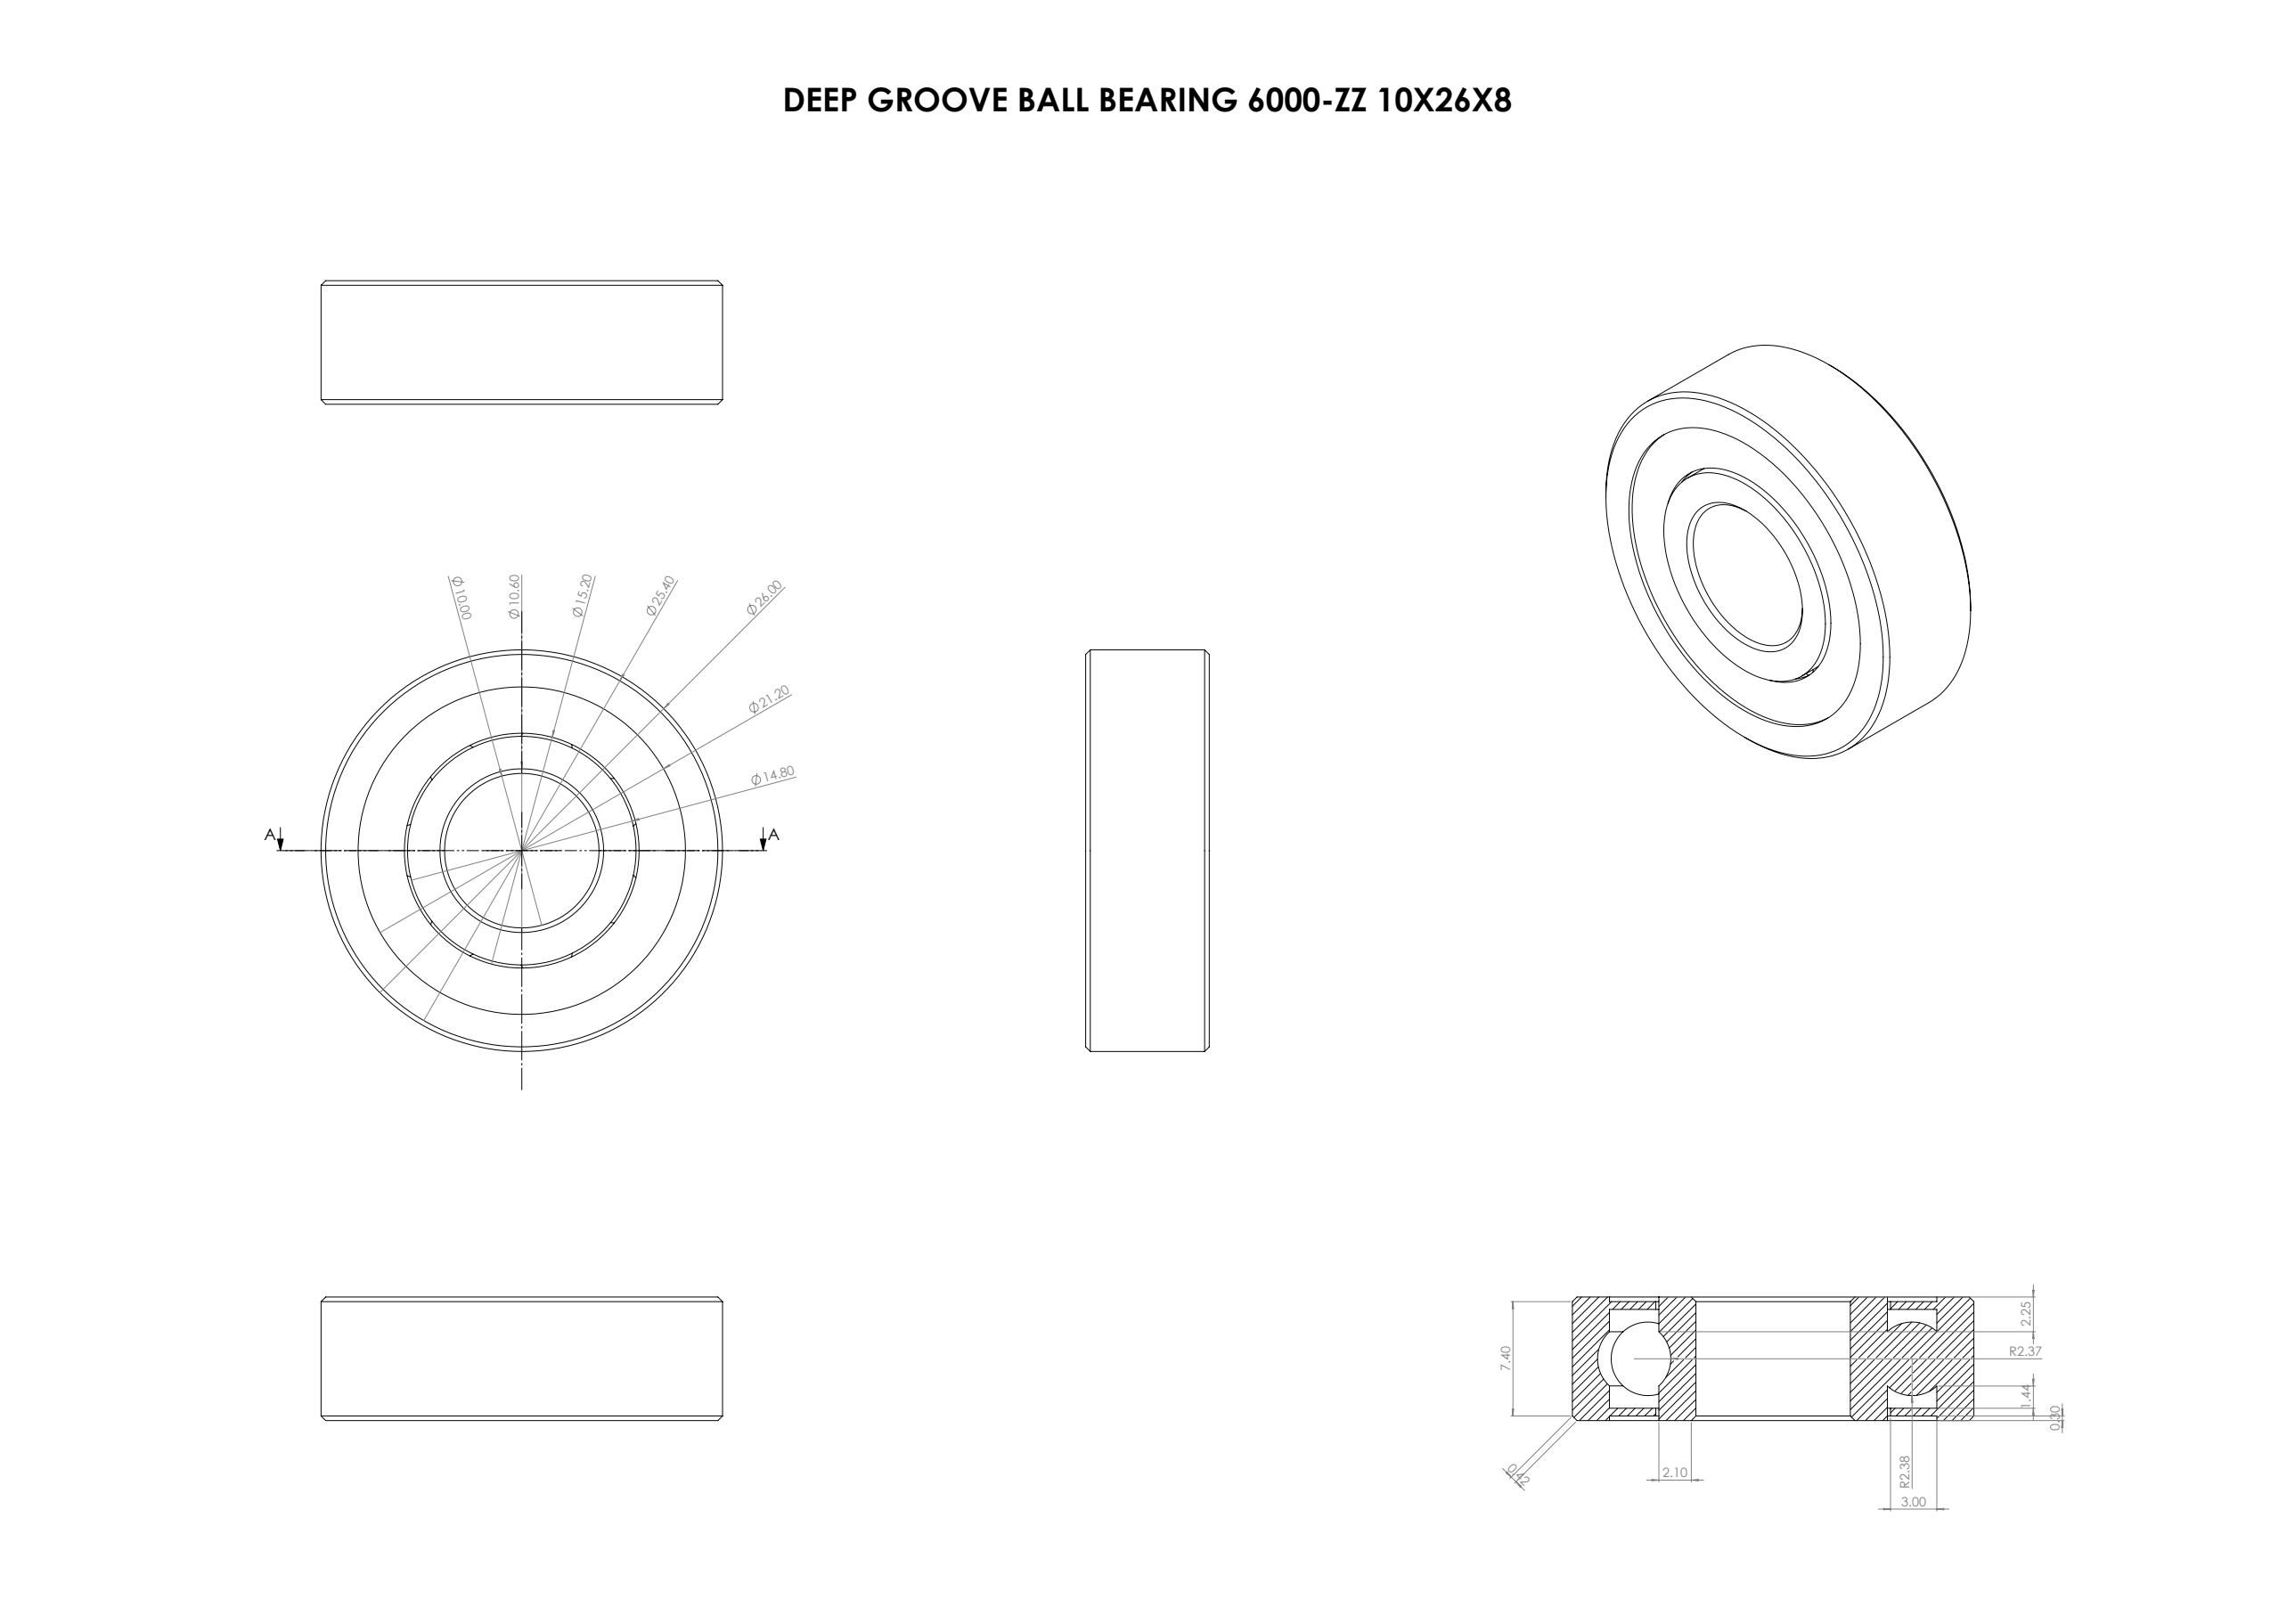
ISO-10303-21;
HEADER;
/* Generated by software containing ST-Developer
 * from STEP Tools, Inc. (www.steptools.com) 
 */

FILE_DESCRIPTION(
/* description */ (''),
/* implementation_level */ '2;1');

FILE_NAME(
/* name */ 
'05_Deep_Groove_Ball_Bearing_6000-ZZ_10x26x8.step',
/* time_stamp */ '2026-10-22T00:21:42-07:00',
/* author */ (''),
/* organization */ (''),
/* preprocessor_version */ 'ST-DEVELOPER v20.2',
/* originating_system */ 'Autodesk Translation Framework v15.15.0.0',
/* authorisation */ '');

FILE_SCHEMA (('AUTOMOTIVE_DESIGN { 1 0 10303 214 3 1 1 }'));
ENDSEC;

DATA;
#10=MECHANICAL_DESIGN_GEOMETRIC_PRESENTATION_REPRESENTATION('',(#209),#31638);
#176=SPHERICAL_SURFACE('',#13012,0.23815);
#177=SPHERICAL_SURFACE('',#13037,0.23815);
#178=SPHERICAL_SURFACE('',#13043,0.23815);
#179=SPHERICAL_SURFACE('',#13050,0.23815);
#180=SPHERICAL_SURFACE('',#13056,0.23815);
#181=SPHERICAL_SURFACE('',#13062,0.23815);
#182=SPHERICAL_SURFACE('',#13073,0.23815);
#187=SHAPE_REPRESENTATION_RELATIONSHIP('SRR','None',#31709,#198);
#198=ADVANCED_BREP_SHAPE_REPRESENTATION('',(#220),#31631);
#209=STYLED_ITEM('',(#31830),#220);
#220=MANIFOLD_SOLID_BREP('6000-ZZ rings + balls + shields',#12484);
#231=TOROIDAL_SURFACE('',#13024,0.9,0.2374);
#232=TOROIDAL_SURFACE('',#13035,0.9,0.2374);
#233=TOROIDAL_SURFACE('',#13040,0.9,0.2374);
#234=TOROIDAL_SURFACE('',#13041,0.9,0.2374);
#235=TOROIDAL_SURFACE('',#13046,0.9,0.2374);
#236=TOROIDAL_SURFACE('',#13047,0.9,0.2374);
#237=TOROIDAL_SURFACE('',#13053,0.9,0.2374);
#238=TOROIDAL_SURFACE('',#13054,0.9,0.2374);
#239=TOROIDAL_SURFACE('',#13059,0.9,0.2374);
#240=TOROIDAL_SURFACE('',#13060,0.9,0.2374);
#241=TOROIDAL_SURFACE('',#13067,0.9,0.2374);
#242=TOROIDAL_SURFACE('',#13072,0.9,0.2374);
#243=TOROIDAL_SURFACE('',#13076,0.9,0.2374);
#244=TOROIDAL_SURFACE('',#13086,0.9,0.2374);
#277=CYLINDRICAL_SURFACE('',#12993,0.76);
#278=CYLINDRICAL_SURFACE('',#12994,1.06);
#279=CYLINDRICAL_SURFACE('',#13002,0.76);
#280=CYLINDRICAL_SURFACE('',#13003,1.06);
#281=CYLINDRICAL_SURFACE('',#13015,1.06);
#282=CYLINDRICAL_SURFACE('',#13025,0.74);
#283=CYLINDRICAL_SURFACE('',#13065,1.06);
#284=CYLINDRICAL_SURFACE('',#13068,0.74);
#285=CYLINDRICAL_SURFACE('',#13081,1.3);
#286=CYLINDRICAL_SURFACE('',#13087,0.5);
#431=CONICAL_SURFACE('',#13079,1.285,0.785398163397452);
#432=CONICAL_SURFACE('',#13083,1.285,0.785398163397452);
#433=CONICAL_SURFACE('',#13090,0.515,0.785398163397452);
#434=CONICAL_SURFACE('',#13095,0.515,0.785398163397452);
#945=B_SPLINE_CURVE_WITH_KNOTS('',3,(#24703,#24704,#24705,#24706,#24707,
#24708),.UNSPECIFIED.,.F.,.F.,(4,2,4),(0.254797907722713,0.274731256245471,
0.294664604768228),.UNSPECIFIED.);
#946=B_SPLINE_CURVE_WITH_KNOTS('',3,(#24712,#24713,#24714,#24715,#24716,
#24717),.UNSPECIFIED.,.F.,.F.,(4,2,4),(0.254797907722713,0.274731256245471,
0.294664604768229),.UNSPECIFIED.);
#947=B_SPLINE_CURVE_WITH_KNOTS('',3,(#24721,#24722,#24723,#24724,#24725,
#24726),.UNSPECIFIED.,.F.,.F.,(4,2,4),(0.254797907722713,0.274731256245471,
0.294664604768229),.UNSPECIFIED.);
#948=B_SPLINE_CURVE_WITH_KNOTS('',3,(#24730,#24731,#24732,#24733,#24734,
#24735),.UNSPECIFIED.,.F.,.F.,(4,2,4),(0.254797907722713,0.274731256245471,
0.294664604768228),.UNSPECIFIED.);
#949=B_SPLINE_CURVE_WITH_KNOTS('',3,(#24739,#24740,#24741,#24742,#24743,
#24744),.UNSPECIFIED.,.F.,.F.,(4,2,4),(0.254797907722728,0.274731256245471,
0.294664604768213),.UNSPECIFIED.);
#950=B_SPLINE_CURVE_WITH_KNOTS('',3,(#24751,#24752,#24753,#24754,#24755,
#24756),.UNSPECIFIED.,.F.,.F.,(4,2,4),(0.254797907722713,0.274731256245471,
0.294664604768229),.UNSPECIFIED.);
#951=B_SPLINE_CURVE_WITH_KNOTS('',3,(#24760,#24761,#24762,#24763,#24764,
#24765),.UNSPECIFIED.,.F.,.F.,(4,2,4),(0.254797907722728,0.274731256245471,
0.294664604768213),.UNSPECIFIED.);
#952=B_SPLINE_CURVE_WITH_KNOTS('',3,(#24770,#24771,#24772,#24773),
 .UNSPECIFIED.,.F.,.F.,(4,4),(0.750997797800867,0.767662411819255),
 .UNSPECIFIED.);
#953=B_SPLINE_CURVE_WITH_KNOTS('',3,(#24775,#24776,#24777,#24778,#24779,
#24780,#24781,#24782,#24783,#24784,#24785,#24786,#24787,#24788,#24789,#24790,
#24791,#24792,#24793,#24794,#24795,#24796),.UNSPECIFIED.,.F.,.F.,(4,2,2,
2,2,2,2,2,2,2,4),(0.516725915130786,0.527390969880923,0.571339243451659,
0.615287517022395,0.659234130021226,0.703180743020057,0.747127356018888,
0.791073969017719,0.835022242588455,0.878970516159191,0.889635570909327),
 .UNSPECIFIED.);
#954=B_SPLINE_CURVE_WITH_KNOTS('',3,(#24798,#24799,#24800,#24801),
 .UNSPECIFIED.,.F.,.F.,(4,4),(0.255887470606418,0.272552084624806),
 .UNSPECIFIED.);
#955=B_SPLINE_CURVE_WITH_KNOTS('',3,(#24805,#24806,#24807,#24808),
 .UNSPECIFIED.,.F.,.F.,(4,4),(0.239222856588031,0.255887470606418),
 .UNSPECIFIED.);
#956=B_SPLINE_CURVE_WITH_KNOTS('',3,(#24810,#24811,#24812,#24813,#24814,
#24815,#24816,#24817,#24818,#24819,#24820,#24821,#24822,#24823,#24824,#24825,
#24826,#24827,#24828,#24829,#24830,#24831),.UNSPECIFIED.,.F.,.F.,(4,2,2,
2,2,2,2,2,2,2,4),(0.516725915130786,0.527390969880923,0.571339243451659,
0.615287517022395,0.659234130021226,0.703180743020057,0.747127356018888,
0.791073969017718,0.835022242588455,0.878970516159191,0.889635570909327),
 .UNSPECIFIED.);
#957=B_SPLINE_CURVE_WITH_KNOTS('',3,(#24832,#24833,#24834,#24835),
 .UNSPECIFIED.,.F.,.F.,(4,4),(0.767662411819255,0.784327025837643),
 .UNSPECIFIED.);
#958=B_SPLINE_CURVE_WITH_KNOTS('',3,(#24839,#24840,#24841,#24842,#24843,
#24844,#24845,#24846,#24847,#24848,#24849,#24850,#24851,#24852,#24853,#24854,
#24855,#24856,#24857,#24858,#24859,#24860,#24861),.UNSPECIFIED.,.F.,.F.,
(4,2,2,2,2,3,2,2,2,2,4),(-0.186453873187253,-0.17578960100413,-0.131841711164795,
-0.087893821325461,-0.0439469106627304,0.,0.0439469106627304,0.0878938213254609,
0.131841711164795,0.17578960100413,0.186453873187381),.UNSPECIFIED.);
#959=B_SPLINE_CURVE_WITH_KNOTS('',3,(#24863,#24864,#24865,#24866,#24867,
#24868),.UNSPECIFIED.,.F.,.F.,(4,2,4),(0.804260420213654,0.824193768736411,
0.844127117259169),.UNSPECIFIED.);
#960=B_SPLINE_CURVE_WITH_KNOTS('',3,(#24869,#24870,#24871,#24872,#24873,
#24874,#24875,#24876,#24877,#24878,#24879,#24880,#24881,#24882,#24883,#24884,
#24885,#24886,#24887,#24888,#24889,#24890,#24891),.UNSPECIFIED.,.F.,.F.,
(4,2,2,2,2,3,2,2,2,2,4),(-0.186453873187253,-0.17578960100413,-0.131841711164795,
-0.087893821325461,-0.0439469106627306,0.,0.0439469106627304,0.0878938213254609,
0.131841711164795,0.17578960100413,0.186453873187381),.UNSPECIFIED.);
#961=B_SPLINE_CURVE_WITH_KNOTS('',3,(#24898,#24899,#24900,#24901,#24902,
#24903),.UNSPECIFIED.,.F.,.F.,(4,2,4),(0.804260420213644,0.824193768736412,
0.84412711725918),.UNSPECIFIED.);
#962=B_SPLINE_CURVE_WITH_KNOTS('',3,(#24907,#24908,#24909,#24910,#24911,
#24912),.UNSPECIFIED.,.F.,.F.,(4,2,4),(0.804260420213654,0.824193768736412,
0.84412711725917),.UNSPECIFIED.);
#963=B_SPLINE_CURVE_WITH_KNOTS('',3,(#24916,#24917,#24918,#24919,#24920,
#24921),.UNSPECIFIED.,.F.,.F.,(4,2,4),(0.804260420213654,0.824193768736411,
0.844127117259169),.UNSPECIFIED.);
#964=B_SPLINE_CURVE_WITH_KNOTS('',3,(#24925,#24926,#24927,#24928,#24929,
#24930),.UNSPECIFIED.,.F.,.F.,(4,2,4),(0.804260420213654,0.824193768736411,
0.844127117259169),.UNSPECIFIED.);
#965=B_SPLINE_CURVE_WITH_KNOTS('',3,(#24935,#24936,#24937,#24938,#24939,
#24940),.UNSPECIFIED.,.F.,.F.,(4,2,4),(0.804260420213643,0.824193768736411,
0.844127117259179),.UNSPECIFIED.);
#966=B_SPLINE_CURVE_WITH_KNOTS('',3,(#24944,#24945,#24946,#24947,#24948,
#24949),.UNSPECIFIED.,.F.,.F.,(4,2,4),(0.804260420213654,0.824193768736412,
0.844127117259169),.UNSPECIFIED.);
#967=B_SPLINE_CURVE_WITH_KNOTS('',3,(#24952,#24953,#24954,#24955,#24956,
#24957,#24958,#24959,#24960,#24961,#24962,#24963,#24964,#24965,#24966,#24967,
#24968,#24969,#24970,#24971,#24972,#24973,#24974),.UNSPECIFIED.,.F.,.F.,
(4,2,2,2,2,3,2,2,2,2,4),(-0.186453873187254,-0.17578960100413,-0.131841711164795,
-0.087893821325461,-0.0439469106627304,0.,0.0439469106627307,0.0878938213254614,
0.131841711164796,0.17578960100413,0.186453873187382),.UNSPECIFIED.);
#968=B_SPLINE_CURVE_WITH_KNOTS('',3,(#24979,#24980,#24981,#24982),
 .UNSPECIFIED.,.F.,.F.,(4,4),(0.23922285658804,0.255887470606418),
 .UNSPECIFIED.);
#969=B_SPLINE_CURVE_WITH_KNOTS('',3,(#24984,#24985,#24986,#24987),
 .UNSPECIFIED.,.F.,.F.,(4,4),(0.255887470606418,0.272552084624797),
 .UNSPECIFIED.);
#970=B_SPLINE_CURVE_WITH_KNOTS('',3,(#24991,#24992,#24993,#24994),
 .UNSPECIFIED.,.F.,.F.,(4,4),(0.239222856588031,0.255887470606418),
 .UNSPECIFIED.);
#971=B_SPLINE_CURVE_WITH_KNOTS('',3,(#24996,#24997,#24998,#24999),
 .UNSPECIFIED.,.F.,.F.,(4,4),(0.255887470606418,0.272552084624806),
 .UNSPECIFIED.);
#972=B_SPLINE_CURVE_WITH_KNOTS('',3,(#25008,#25009,#25010,#25011),
 .UNSPECIFIED.,.F.,.F.,(4,4),(0.239222856588039,0.255887470606418),
 .UNSPECIFIED.);
#973=B_SPLINE_CURVE_WITH_KNOTS('',3,(#25013,#25014,#25015,#25016),
 .UNSPECIFIED.,.F.,.F.,(4,4),(0.255887470606418,0.272552084624797),
 .UNSPECIFIED.);
#974=B_SPLINE_CURVE_WITH_KNOTS('',3,(#25020,#25021,#25022,#25023),
 .UNSPECIFIED.,.F.,.F.,(4,4),(0.239222856588031,0.255887470606418),
 .UNSPECIFIED.);
#975=B_SPLINE_CURVE_WITH_KNOTS('',3,(#25025,#25026,#25027,#25028),
 .UNSPECIFIED.,.F.,.F.,(4,4),(0.255887470606418,0.272552084624806),
 .UNSPECIFIED.);
#976=B_SPLINE_CURVE_WITH_KNOTS('',3,(#25032,#25033,#25034,#25035),
 .UNSPECIFIED.,.F.,.F.,(4,4),(0.239222856588031,0.255887470606418),
 .UNSPECIFIED.);
#977=B_SPLINE_CURVE_WITH_KNOTS('',3,(#25037,#25038,#25039,#25040),
 .UNSPECIFIED.,.F.,.F.,(4,4),(0.255887470606418,0.272552084624806),
 .UNSPECIFIED.);
#978=B_SPLINE_CURVE_WITH_KNOTS('',3,(#25044,#25045,#25046,#25047),
 .UNSPECIFIED.,.F.,.F.,(4,4),(0.239222856588031,0.255887470606418),
 .UNSPECIFIED.);
#979=B_SPLINE_CURVE_WITH_KNOTS('',3,(#25049,#25050,#25051,#25052),
 .UNSPECIFIED.,.F.,.F.,(4,4),(0.255887470606418,0.272552084624806),
 .UNSPECIFIED.);
#980=B_SPLINE_CURVE_WITH_KNOTS('',3,(#25057,#25058,#25059,#25060,#25061,
#25062,#25063,#25064,#25065,#25066,#25067,#25068,#25069,#25070,#25071,#25072,
#25073,#25074,#25075,#25076,#25077,#25078),.UNSPECIFIED.,.F.,.F.,(4,2,2,
2,2,2,2,2,2,2,4),(0.516725915130786,0.527390969880923,0.571339243451659,
0.615287517022395,0.659234130021226,0.703180743020057,0.747127356018888,
0.791073969017719,0.835022242588455,0.878970516159191,0.889635570909327),
 .UNSPECIFIED.);
#981=B_SPLINE_CURVE_WITH_KNOTS('',3,(#25082,#25083,#25084,#25085),
 .UNSPECIFIED.,.F.,.F.,(4,4),(0.750997797800864,0.767662411819255),
 .UNSPECIFIED.);
#982=B_SPLINE_CURVE_WITH_KNOTS('',3,(#25086,#25087,#25088,#25089,#25090,
#25091,#25092,#25093,#25094,#25095,#25096,#25097,#25098,#25099,#25100,#25101,
#25102,#25103,#25104,#25105,#25106,#25107),.UNSPECIFIED.,.F.,.F.,(4,2,2,
2,2,2,2,2,2,2,4),(0.516725915130786,0.527390969880923,0.571339243451659,
0.615287517022395,0.659234130021226,0.703180743020056,0.747127356018887,
0.791073969017719,0.835022242588454,0.87897051615919,0.889635570909327),
 .UNSPECIFIED.);
#983=B_SPLINE_CURVE_WITH_KNOTS('',3,(#25110,#25111,#25112,#25113),
 .UNSPECIFIED.,.F.,.F.,(4,4),(0.767662411819255,0.784327025837645),
 .UNSPECIFIED.);
#984=B_SPLINE_CURVE_WITH_KNOTS('',3,(#25116,#25117,#25118,#25119,#25120,
#25121,#25122,#25123,#25124,#25125,#25126,#25127,#25128,#25129,#25130,#25131,
#25132,#25133,#25134,#25135,#25136,#25137,#25138),.UNSPECIFIED.,.F.,.F.,
(4,2,2,2,2,3,2,2,2,2,4),(-0.186453873187254,-0.17578960100413,-0.131841711164796,
-0.0878938213254614,-0.0439469106627306,0.,0.0439469106627305,0.0878938213254609,
0.131841711164795,0.175789601004129,0.186453873187382),.UNSPECIFIED.);
#985=B_SPLINE_CURVE_WITH_KNOTS('',3,(#25140,#25141,#25142,#25143,#25144,
#25145,#25146,#25147,#25148,#25149,#25150,#25151,#25152,#25153,#25154,#25155,
#25156,#25157,#25158,#25159,#25160,#25161,#25162),.UNSPECIFIED.,.F.,.F.,
(4,2,2,2,2,3,2,2,2,2,4),(-0.186453873187253,-0.17578960100413,-0.131841711164795,
-0.087893821325461,-0.0439469106627306,0.,0.0439469106627305,0.0878938213254609,
0.131841711164795,0.17578960100413,0.186453873187381),.UNSPECIFIED.);
#986=B_SPLINE_CURVE_WITH_KNOTS('',3,(#25166,#25167,#25168,#25169,#25170,
#25171,#25172,#25173,#25174,#25175,#25176,#25177,#25178,#25179,#25180,#25181,
#25182,#25183,#25184,#25185,#25186,#25187),.UNSPECIFIED.,.F.,.F.,(4,2,2,
2,2,2,2,2,2,2,4),(0.516725915130786,0.527390969880923,0.571339243451659,
0.615287517022395,0.659234130021226,0.703180743020057,0.747127356018888,
0.791073969017718,0.835022242588455,0.878970516159191,0.889635570909327),
 .UNSPECIFIED.);
#987=B_SPLINE_CURVE_WITH_KNOTS('',3,(#25191,#25192,#25193,#25194),
 .UNSPECIFIED.,.F.,.F.,(4,4),(0.750997797800867,0.767662411819255),
 .UNSPECIFIED.);
#988=B_SPLINE_CURVE_WITH_KNOTS('',3,(#25195,#25196,#25197,#25198,#25199,
#25200,#25201,#25202,#25203,#25204,#25205,#25206,#25207,#25208,#25209,#25210,
#25211,#25212,#25213,#25214,#25215,#25216),.UNSPECIFIED.,.F.,.F.,(4,2,2,
2,2,2,2,2,2,2,4),(0.516725915130786,0.527390969880923,0.571339243451659,
0.615287517022395,0.659234130021226,0.703180743020057,0.747127356018888,
0.791073969017718,0.835022242588454,0.87897051615919,0.889635570909327),
 .UNSPECIFIED.);
#989=B_SPLINE_CURVE_WITH_KNOTS('',3,(#25219,#25220,#25221,#25222),
 .UNSPECIFIED.,.F.,.F.,(4,4),(0.767662411819255,0.784327025837642),
 .UNSPECIFIED.);
#990=B_SPLINE_CURVE_WITH_KNOTS('',3,(#25225,#25226,#25227,#25228,#25229,
#25230,#25231,#25232,#25233,#25234,#25235,#25236,#25237,#25238,#25239,#25240,
#25241,#25242,#25243,#25244,#25245,#25246,#25247),.UNSPECIFIED.,.F.,.F.,
(4,2,2,2,2,3,2,2,2,2,4),(-0.186453873187253,-0.17578960100413,-0.131841711164795,
-0.0878938213254608,-0.0439469106627304,0.,0.0439469106627304,0.0878938213254609,
0.131841711164795,0.17578960100413,0.186453873187381),.UNSPECIFIED.);
#991=B_SPLINE_CURVE_WITH_KNOTS('',3,(#25249,#25250,#25251,#25252,#25253,
#25254,#25255,#25256,#25257,#25258,#25259,#25260,#25261,#25262,#25263,#25264,
#25265,#25266,#25267,#25268,#25269,#25270,#25271),.UNSPECIFIED.,.F.,.F.,
(4,2,2,2,2,3,2,2,2,2,4),(-0.186453873187254,-0.17578960100413,-0.131841711164796,
-0.0878938213254614,-0.0439469106627308,0.,0.0439469106627309,0.0878938213254618,
0.131841711164796,0.17578960100413,0.186453873187382),.UNSPECIFIED.);
#992=B_SPLINE_CURVE_WITH_KNOTS('',3,(#25277,#25278,#25279,#25280,#25281,
#25282,#25283,#25284,#25285,#25286,#25287,#25288,#25289,#25290,#25291,#25292,
#25293,#25294,#25295,#25296,#25297,#25298),.UNSPECIFIED.,.F.,.F.,(4,2,2,
2,2,2,2,2,2,2,4),(0.516725915130787,0.527390969880924,0.571339243451659,
0.615287517022395,0.659234130021226,0.703180743020058,0.747127356018888,
0.791073969017719,0.835022242588455,0.878970516159191,0.889635570909328),
 .UNSPECIFIED.);
#993=B_SPLINE_CURVE_WITH_KNOTS('',3,(#25302,#25303,#25304,#25305),
 .UNSPECIFIED.,.F.,.F.,(4,4),(0.750997797800863,0.767662411819254),
 .UNSPECIFIED.);
#994=B_SPLINE_CURVE_WITH_KNOTS('',3,(#25306,#25307,#25308,#25309,#25310,
#25311,#25312,#25313,#25314,#25315,#25316,#25317,#25318,#25319,#25320,#25321,
#25322,#25323,#25324,#25325,#25326,#25327),.UNSPECIFIED.,.F.,.F.,(4,2,2,
2,2,2,2,2,2,2,4),(0.516725915130786,0.527390969880923,0.571339243451659,
0.615287517022395,0.659234130021226,0.703180743020056,0.747127356018888,
0.791073969017719,0.835022242588455,0.87897051615919,0.889635570909327),
 .UNSPECIFIED.);
#995=B_SPLINE_CURVE_WITH_KNOTS('',3,(#25330,#25331,#25332,#25333),
 .UNSPECIFIED.,.F.,.F.,(4,4),(0.767662411819254,0.784327025837645),
 .UNSPECIFIED.);
#996=B_SPLINE_CURVE_WITH_KNOTS('',3,(#25336,#25337,#25338,#25339,#25340,
#25341,#25342,#25343,#25344,#25345,#25346,#25347,#25348,#25349,#25350,#25351,
#25352,#25353,#25354,#25355,#25356,#25357,#25358),.UNSPECIFIED.,.F.,.F.,
(4,2,2,2,2,3,2,2,2,2,4),(-0.186453873187254,-0.17578960100413,-0.131841711164796,
-0.0878938213254616,-0.0439469106627308,0.,0.0439469106627307,0.0878938213254613,
0.131841711164795,0.17578960100413,0.186453873187382),.UNSPECIFIED.);
#997=B_SPLINE_CURVE_WITH_KNOTS('',3,(#25360,#25361,#25362,#25363,#25364,
#25365,#25366,#25367,#25368,#25369,#25370,#25371,#25372,#25373,#25374,#25375,
#25376,#25377,#25378,#25379,#25380,#25381,#25382),.UNSPECIFIED.,.F.,.F.,
(4,2,2,2,2,3,2,2,2,2,4),(-0.186453873187253,-0.17578960100413,-0.131841711164795,
-0.0878938213254608,-0.0439469106627304,0.,0.0439469106627304,0.0878938213254609,
0.131841711164795,0.17578960100413,0.186453873187382),.UNSPECIFIED.);
#998=B_SPLINE_CURVE_WITH_KNOTS('',3,(#25386,#25387,#25388,#25389,#25390,
#25391,#25392,#25393,#25394,#25395,#25396,#25397,#25398,#25399,#25400,#25401,
#25402,#25403,#25404,#25405,#25406,#25407),.UNSPECIFIED.,.F.,.F.,(4,2,2,
2,2,2,2,2,2,2,4),(0.516725915130786,0.527390969880923,0.571339243451659,
0.615287517022395,0.659234130021226,0.703180743020057,0.747127356018888,
0.791073969017719,0.835022242588455,0.878970516159191,0.889635570909327),
 .UNSPECIFIED.);
#999=B_SPLINE_CURVE_WITH_KNOTS('',3,(#25411,#25412,#25413,#25414),
 .UNSPECIFIED.,.F.,.F.,(4,4),(0.750997797800867,0.767662411819255),
 .UNSPECIFIED.);
#1000=B_SPLINE_CURVE_WITH_KNOTS('',3,(#25415,#25416,#25417,#25418,#25419,
#25420,#25421,#25422,#25423,#25424,#25425,#25426,#25427,#25428,#25429,#25430,
#25431,#25432,#25433,#25434,#25435,#25436),.UNSPECIFIED.,.F.,.F.,(4,2,2,
2,2,2,2,2,2,2,4),(0.516725915130786,0.527390969880923,0.571339243451659,
0.615287517022395,0.659234130021226,0.703180743020057,0.747127356018888,
0.791073969017718,0.835022242588454,0.87897051615919,0.889635570909327),
 .UNSPECIFIED.);
#1001=B_SPLINE_CURVE_WITH_KNOTS('',3,(#25439,#25440,#25441,#25442),
 .UNSPECIFIED.,.F.,.F.,(4,4),(0.767662411819255,0.784327025837643),
 .UNSPECIFIED.);
#1002=B_SPLINE_CURVE_WITH_KNOTS('',3,(#25445,#25446,#25447,#25448,#25449,
#25450,#25451,#25452,#25453,#25454,#25455,#25456,#25457,#25458,#25459,#25460,
#25461,#25462,#25463,#25464,#25465,#25466,#25467),.UNSPECIFIED.,.F.,.F.,
(4,2,2,2,2,3,2,2,2,2,4),(-0.186453873187253,-0.17578960100413,-0.131841711164795,
-0.0878938213254608,-0.0439469106627304,0.,0.0439469106627304,0.0878938213254608,
0.131841711164795,0.17578960100413,0.186453873187381),.UNSPECIFIED.);
#1003=B_SPLINE_CURVE_WITH_KNOTS('',3,(#25469,#25470,#25471,#25472,#25473,
#25474,#25475,#25476,#25477,#25478,#25479,#25480,#25481,#25482,#25483,#25484,
#25485,#25486,#25487,#25488,#25489,#25490,#25491),.UNSPECIFIED.,.F.,.F.,
(4,2,2,2,2,3,2,2,2,2,4),(-0.186453873187253,-0.17578960100413,-0.131841711164796,
-0.0878938213254616,-0.0439469106627308,0.,0.0439469106627304,0.0878938213254609,
0.131841711164795,0.17578960100413,0.186453873187382),.UNSPECIFIED.);
#1004=B_SPLINE_CURVE_WITH_KNOTS('',3,(#25495,#25496,#25497,#25498,#25499,
#25500,#25501,#25502,#25503,#25504,#25505,#25506,#25507,#25508,#25509,#25510,
#25511,#25512,#25513,#25514,#25515,#25516),.UNSPECIFIED.,.F.,.F.,(4,2,2,
2,2,2,2,2,2,2,4),(0.516725915130786,0.527390969880923,0.571339243451659,
0.615287517022395,0.659234130021226,0.703180743020057,0.747127356018888,
0.791073969017719,0.835022242588455,0.878970516159191,0.889635570909328),
 .UNSPECIFIED.);
#1005=B_SPLINE_CURVE_WITH_KNOTS('',3,(#25519,#25520,#25521,#25522),
 .UNSPECIFIED.,.F.,.F.,(4,4),(0.767662411819255,0.784327025837642),
 .UNSPECIFIED.);
#1006=B_SPLINE_CURVE_WITH_KNOTS('',3,(#25526,#25527,#25528,#25529),
 .UNSPECIFIED.,.F.,.F.,(4,4),(0.750997797800867,0.767662411819255),
 .UNSPECIFIED.);
#1007=B_SPLINE_CURVE_WITH_KNOTS('',3,(#25530,#25531,#25532,#25533,#25534,
#25535,#25536,#25537,#25538,#25539,#25540,#25541,#25542,#25543,#25544,#25545,
#25546,#25547,#25548,#25549,#25550,#25551),.UNSPECIFIED.,.F.,.F.,(4,2,2,
2,2,2,2,2,2,2,4),(0.516725915130786,0.527390969880923,0.571339243451659,
0.615287517022395,0.659234130021226,0.703180743020057,0.747127356018888,
0.791073969017719,0.835022242588455,0.878970516159191,0.889635570909327),
 .UNSPECIFIED.);
#1008=B_SPLINE_CURVE_WITH_KNOTS('',3,(#25554,#25555,#25556,#25557,#25558,
#25559,#25560,#25561,#25562,#25563,#25564,#25565,#25566,#25567,#25568,#25569,
#25570,#25571,#25572,#25573,#25574,#25575,#25576),.UNSPECIFIED.,.F.,.F.,
(4,2,2,2,2,3,2,2,2,2,4),(-0.186453873187254,-0.17578960100413,-0.131841711164795,
-0.087893821325461,-0.0439469106627304,0.,0.0439469106627308,0.0878938213254617,
0.131841711164796,0.17578960100413,0.186453873187381),.UNSPECIFIED.);
#1009=B_SPLINE_CURVE_WITH_KNOTS('',3,(#25582,#25583,#25584,#25585,#25586,
#25587,#25588,#25589,#25590,#25591,#25592,#25593,#25594,#25595,#25596,#25597,
#25598,#25599,#25600,#25601,#25602,#25603,#25604),.UNSPECIFIED.,.F.,.F.,
(4,2,2,2,2,3,2,2,2,2,4),(-0.186453873187253,-0.17578960100413,-0.131841711164795,
-0.0878938213254608,-0.0439469106627304,0.,0.0439469106627304,0.0878938213254609,
0.131841711164795,0.17578960100413,0.186453873187381),.UNSPECIFIED.);
#1010=B_SPLINE_CURVE_WITH_KNOTS('',3,(#25612,#25613,#25614,#25615),
 .UNSPECIFIED.,.F.,.F.,(4,4),(0.750997797800867,0.767662411819255),
 .UNSPECIFIED.);
#1011=B_SPLINE_CURVE_WITH_KNOTS('',3,(#25617,#25618,#25619,#25620),
 .UNSPECIFIED.,.F.,.F.,(4,4),(0.767662411819255,0.784327025837643),
 .UNSPECIFIED.);
#1012=B_SPLINE_CURVE_WITH_KNOTS('',3,(#25623,#25624,#25625,#25626,#25627,
#25628,#25629,#25630,#25631,#25632,#25633,#25634,#25635,#25636,#25637,#25638,
#25639,#25640,#25641,#25642,#25643,#25644),.UNSPECIFIED.,.F.,.F.,(4,2,2,
2,2,2,2,2,2,2,4),(0.516725915130786,0.527390969880923,0.571339243451659,
0.615287517022395,0.659234130021226,0.703180743020057,0.747127356018888,
0.791073969017719,0.835022242588455,0.878970516159191,0.889635570909328),
 .UNSPECIFIED.);
#1013=B_SPLINE_CURVE_WITH_KNOTS('',3,(#25648,#25649,#25650,#25651,#25652,
#25653,#25654,#25655,#25656,#25657,#25658,#25659,#25660,#25661,#25662,#25663,
#25664,#25665,#25666,#25667,#25668,#25669),.UNSPECIFIED.,.F.,.F.,(4,2,2,
2,2,2,2,2,2,2,4),(0.516725915130786,0.527390969880923,0.571339243451659,
0.615287517022395,0.659234130021226,0.703180743020057,0.747127356018888,
0.791073969017719,0.835022242588455,0.878970516159191,0.889635570909327),
 .UNSPECIFIED.);
#1014=B_SPLINE_CURVE_WITH_KNOTS('',3,(#25672,#25673,#25674,#25675,#25676,
#25677,#25678,#25679,#25680,#25681,#25682,#25683,#25684,#25685,#25686,#25687,
#25688,#25689,#25690,#25691,#25692,#25693,#25694),.UNSPECIFIED.,.F.,.F.,
(4,2,2,2,2,3,2,2,2,2,4),(-0.186453873187253,-0.17578960100413,-0.131841711164795,
-0.087893821325461,-0.0439469106627306,0.,0.0439469106627304,0.0878938213254609,
0.131841711164795,0.17578960100413,0.186453873187381),.UNSPECIFIED.);
#1375=FACE_BOUND('',#2887,.T.);
#1376=FACE_BOUND('',#2889,.T.);
#1377=FACE_BOUND('',#2893,.T.);
#1378=FACE_BOUND('',#2895,.T.);
#1379=FACE_BOUND('',#2899,.T.);
#1380=FACE_BOUND('',#2905,.T.);
#1381=FACE_BOUND('',#2909,.T.);
#1382=FACE_BOUND('',#2913,.T.);
#1383=FACE_BOUND('',#2917,.T.);
#1384=FACE_BOUND('',#2921,.T.);
#1385=FACE_BOUND('',#2927,.T.);
#1386=FACE_BOUND('',#2930,.T.);
#1387=FACE_BOUND('',#2935,.T.);
#1388=FACE_BOUND('',#2940,.T.);
#1389=FACE_BOUND('',#2942,.T.);
#1579=CIRCLE('',#12988,1.06);
#1580=CIRCLE('',#12989,0.76);
#1581=CIRCLE('',#12991,1.06);
#1582=CIRCLE('',#12992,0.76);
#1583=CIRCLE('',#12995,1.06);
#1584=CIRCLE('',#12997,1.06);
#1585=CIRCLE('',#12998,0.76);
#1586=CIRCLE('',#13000,1.06);
#1587=CIRCLE('',#13001,0.76);
#1588=CIRCLE('',#13004,1.06);
#1589=CIRCLE('',#13005,1.06);
#1590=CIRCLE('',#13006,1.06);
#1591=CIRCLE('',#13007,1.06);
#1592=CIRCLE('',#13008,1.06);
#1593=CIRCLE('',#13009,1.06);
#1594=CIRCLE('',#13010,1.06);
#1595=CIRCLE('',#13011,1.06);
#1596=CIRCLE('',#13013,0.23815);
#1597=CIRCLE('',#13014,0.23815);
#1598=CIRCLE('',#13016,1.06);
#1599=CIRCLE('',#13017,1.06);
#1600=CIRCLE('',#13018,1.06);
#1601=CIRCLE('',#13019,1.06);
#1602=CIRCLE('',#13020,1.06);
#1603=CIRCLE('',#13021,1.06);
#1604=CIRCLE('',#13022,1.06);
#1605=CIRCLE('',#13023,1.06);
#1606=CIRCLE('',#13026,0.74);
#1607=CIRCLE('',#13027,0.74);
#1608=CIRCLE('',#13028,0.74);
#1609=CIRCLE('',#13029,0.74);
#1610=CIRCLE('',#13030,0.74);
#1611=CIRCLE('',#13031,0.74);
#1612=CIRCLE('',#13032,0.74);
#1613=CIRCLE('',#13033,0.74);
#1614=CIRCLE('',#13034,0.74);
#1615=CIRCLE('',#13036,0.74);
#1616=CIRCLE('',#13038,0.23815);
#1617=CIRCLE('',#13039,0.23815);
#1618=CIRCLE('',#13042,0.74);
#1619=CIRCLE('',#13044,0.23815);
#1620=CIRCLE('',#13045,0.23815);
#1621=CIRCLE('',#13048,0.74);
#1622=CIRCLE('',#13049,0.74);
#1623=CIRCLE('',#13051,0.23815);
#1624=CIRCLE('',#13052,0.23815);
#1625=CIRCLE('',#13055,0.74);
#1626=CIRCLE('',#13057,0.23815);
#1627=CIRCLE('',#13058,0.23815);
#1628=CIRCLE('',#13061,0.74);
#1629=CIRCLE('',#13063,0.23815);
#1630=CIRCLE('',#13064,0.23815);
#1631=CIRCLE('',#13066,1.06);
#1632=CIRCLE('',#13069,0.74);
#1633=CIRCLE('',#13070,0.74);
#1634=CIRCLE('',#13071,0.74);
#1635=CIRCLE('',#13074,0.23815);
#1636=CIRCLE('',#13075,0.23815);
#1637=CIRCLE('',#13078,1.27);
#1638=CIRCLE('',#13080,1.3);
#1639=CIRCLE('',#13082,1.3);
#1640=CIRCLE('',#13084,1.27);
#1641=CIRCLE('',#13088,0.5);
#1642=CIRCLE('',#13089,0.5);
#1643=CIRCLE('',#13091,0.53);
#1644=CIRCLE('',#13094,0.53);
#2157=FACE_OUTER_BOUND('',#2886,.T.);
#2158=FACE_OUTER_BOUND('',#2888,.T.);
#2159=FACE_OUTER_BOUND('',#2890,.T.);
#2160=FACE_OUTER_BOUND('',#2891,.T.);
#2161=FACE_OUTER_BOUND('',#2892,.T.);
#2162=FACE_OUTER_BOUND('',#2894,.T.);
#2163=FACE_OUTER_BOUND('',#2896,.T.);
#2164=FACE_OUTER_BOUND('',#2897,.T.);
#2165=FACE_OUTER_BOUND('',#2898,.T.);
#2166=FACE_OUTER_BOUND('',#2900,.T.);
#2167=FACE_OUTER_BOUND('',#2901,.T.);
#2168=FACE_OUTER_BOUND('',#2902,.T.);
#2169=FACE_OUTER_BOUND('',#2903,.T.);
#2170=FACE_OUTER_BOUND('',#2904,.T.);
#2171=FACE_OUTER_BOUND('',#2906,.T.);
#2172=FACE_OUTER_BOUND('',#2907,.T.);
#2173=FACE_OUTER_BOUND('',#2908,.T.);
#2174=FACE_OUTER_BOUND('',#2910,.T.);
#2175=FACE_OUTER_BOUND('',#2911,.T.);
#2176=FACE_OUTER_BOUND('',#2912,.T.);
#2177=FACE_OUTER_BOUND('',#2914,.T.);
#2178=FACE_OUTER_BOUND('',#2915,.T.);
#2179=FACE_OUTER_BOUND('',#2916,.T.);
#2180=FACE_OUTER_BOUND('',#2918,.T.);
#2181=FACE_OUTER_BOUND('',#2919,.T.);
#2182=FACE_OUTER_BOUND('',#2920,.T.);
#2183=FACE_OUTER_BOUND('',#2922,.T.);
#2184=FACE_OUTER_BOUND('',#2923,.T.);
#2185=FACE_OUTER_BOUND('',#2924,.T.);
#2186=FACE_OUTER_BOUND('',#2925,.T.);
#2187=FACE_OUTER_BOUND('',#2926,.T.);
#2188=FACE_OUTER_BOUND('',#2928,.T.);
#2189=FACE_OUTER_BOUND('',#2929,.T.);
#2190=FACE_OUTER_BOUND('',#2931,.T.);
#2191=FACE_OUTER_BOUND('',#2932,.T.);
#2192=FACE_OUTER_BOUND('',#2933,.T.);
#2193=FACE_OUTER_BOUND('',#2934,.T.);
#2194=FACE_OUTER_BOUND('',#2936,.T.);
#2195=FACE_OUTER_BOUND('',#2937,.T.);
#2196=FACE_OUTER_BOUND('',#2938,.T.);
#2197=FACE_OUTER_BOUND('',#2939,.T.);
#2198=FACE_OUTER_BOUND('',#2941,.T.);
#2199=FACE_OUTER_BOUND('',#2943,.T.);
#2886=EDGE_LOOP('',(#9609));
#2887=EDGE_LOOP('',(#9610));
#2888=EDGE_LOOP('',(#9611));
#2889=EDGE_LOOP('',(#9612));
#2890=EDGE_LOOP('',(#9613,#9614,#9615,#9616));
#2891=EDGE_LOOP('',(#9617,#9618,#9619,#9620));
#2892=EDGE_LOOP('',(#9621));
#2893=EDGE_LOOP('',(#9622));
#2894=EDGE_LOOP('',(#9623));
#2895=EDGE_LOOP('',(#9624));
#2896=EDGE_LOOP('',(#9625,#9626,#9627,#9628));
#2897=EDGE_LOOP('',(#9629,#9630,#9631,#9632,#9633,#9634,#9635,#9636,#9637,
#9638,#9639,#9640,#9641,#9642,#9643,#9644,#9645,#9646));
#2898=EDGE_LOOP('',(#9647,#9648,#9649,#9650,#9651,#9652,#9653,#9654,#9655,
#9656));
#2899=EDGE_LOOP('',(#9657,#9658,#9659,#9660));
#2900=EDGE_LOOP('',(#9661,#9662,#9663,#9664,#9665,#9666,#9667,#9668,#9669,
#9670,#9671,#9672,#9673,#9674,#9675,#9676,#9677,#9678));
#2901=EDGE_LOOP('',(#9679,#9680,#9681,#9682));
#2902=EDGE_LOOP('',(#9683,#9684,#9685,#9686,#9687,#9688,#9689,#9690,#9691,
#9692,#9693,#9694,#9695,#9696,#9697,#9698,#9699,#9700,#9701,#9702,#9703,
#9704,#9705,#9706,#9707));
#2903=EDGE_LOOP('',(#9708,#9709,#9710,#9711));
#2904=EDGE_LOOP('',(#9712,#9713,#9714,#9715,#9716,#9717,#9718,#9719,#9720,
#9721));
#2905=EDGE_LOOP('',(#9722,#9723,#9724,#9725));
#2906=EDGE_LOOP('',(#9726,#9727,#9728,#9729));
#2907=EDGE_LOOP('',(#9730,#9731,#9732,#9733));
#2908=EDGE_LOOP('',(#9734,#9735,#9736,#9737,#9738,#9739,#9740,#9741,#9742,
#9743));
#2909=EDGE_LOOP('',(#9744,#9745,#9746,#9747));
#2910=EDGE_LOOP('',(#9748,#9749,#9750,#9751,#9752,#9753));
#2911=EDGE_LOOP('',(#9754,#9755,#9756,#9757,#9758,#9759));
#2912=EDGE_LOOP('',(#9760,#9761,#9762,#9763,#9764,#9765,#9766,#9767,#9768,
#9769));
#2913=EDGE_LOOP('',(#9770,#9771,#9772,#9773));
#2914=EDGE_LOOP('',(#9774,#9775,#9776,#9777));
#2915=EDGE_LOOP('',(#9778,#9779,#9780,#9781));
#2916=EDGE_LOOP('',(#9782,#9783,#9784,#9785,#9786,#9787,#9788,#9789,#9790,
#9791));
#2917=EDGE_LOOP('',(#9792,#9793,#9794,#9795));
#2918=EDGE_LOOP('',(#9796,#9797,#9798,#9799));
#2919=EDGE_LOOP('',(#9800,#9801,#9802,#9803));
#2920=EDGE_LOOP('',(#9804,#9805,#9806,#9807,#9808,#9809,#9810,#9811,#9812,
#9813));
#2921=EDGE_LOOP('',(#9814,#9815,#9816,#9817));
#2922=EDGE_LOOP('',(#9818,#9819,#9820,#9821));
#2923=EDGE_LOOP('',(#9822,#9823,#9824,#9825));
#2924=EDGE_LOOP('',(#9826,#9827,#9828,#9829,#9830,#9831,#9832,#9833,#9834,
#9835,#9836,#9837,#9838,#9839,#9840,#9841,#9842,#9843,#9844,#9845,#9846,
#9847,#9848,#9849,#9850));
#2925=EDGE_LOOP('',(#9851,#9852,#9853,#9854));
#2926=EDGE_LOOP('',(#9855,#9856,#9857,#9858,#9859,#9860,#9861,#9862,#9863,
#9864));
#2927=EDGE_LOOP('',(#9865,#9866,#9867,#9868));
#2928=EDGE_LOOP('',(#9869,#9870,#9871,#9872));
#2929=EDGE_LOOP('',(#9873));
#2930=EDGE_LOOP('',(#9874));
#2931=EDGE_LOOP('',(#9875,#9876,#9877,#9878));
#2932=EDGE_LOOP('',(#9879,#9880,#9881,#9882));
#2933=EDGE_LOOP('',(#9883,#9884,#9885,#9886));
#2934=EDGE_LOOP('',(#9887));
#2935=EDGE_LOOP('',(#9888));
#2936=EDGE_LOOP('',(#9889,#9890,#9891,#9892));
#2937=EDGE_LOOP('',(#9893,#9894,#9895,#9896));
#2938=EDGE_LOOP('',(#9897,#9898,#9899,#9900));
#2939=EDGE_LOOP('',(#9901));
#2940=EDGE_LOOP('',(#9902));
#2941=EDGE_LOOP('',(#9903));
#2942=EDGE_LOOP('',(#9904));
#2943=EDGE_LOOP('',(#9905,#9906,#9907,#9908));
#3538=LINE('',#24683,#4243);
#3539=LINE('',#24687,#4244);
#3540=LINE('',#24699,#4245);
#3541=LINE('',#24747,#4246);
#3542=LINE('',#24894,#4247);
#3543=LINE('',#25003,#4248);
#3544=LINE('',#25579,#4249);
#3545=LINE('',#25608,#4250);
#3546=LINE('',#25702,#4251);
#3547=LINE('',#25706,#4252);
#3548=LINE('',#25710,#4253);
#3549=LINE('',#25717,#4254);
#3550=LINE('',#25721,#4255);
#3551=LINE('',#25728,#4256);
#4243=VECTOR('',#14648,0.76);
#4244=VECTOR('',#14653,1.06);
#4245=VECTOR('',#14668,0.76);
#4246=VECTOR('',#14681,1.06);
#4247=VECTOR('',#14696,1.06);
#4248=VECTOR('',#14723,0.74);
#4249=VECTOR('',#14798,1.06);
#4250=VECTOR('',#14807,0.74);
#4251=VECTOR('',#14830,1.285);
#4252=VECTOR('',#14835,1.3);
#4253=VECTOR('',#14840,1.285);
#4254=VECTOR('',#14849,0.5);
#4255=VECTOR('',#14854,0.515);
#4256=VECTOR('',#14865,0.515);
#5289=VERTEX_POINT('',#24673);
#5290=VERTEX_POINT('',#24675);
#5291=VERTEX_POINT('',#24678);
#5292=VERTEX_POINT('',#24680);
#5293=VERTEX_POINT('',#24685);
#5294=VERTEX_POINT('',#24689);
#5295=VERTEX_POINT('',#24691);
#5296=VERTEX_POINT('',#24694);
#5297=VERTEX_POINT('',#24696);
#5298=VERTEX_POINT('',#24701);
#5299=VERTEX_POINT('',#24702);
#5300=VERTEX_POINT('',#24709);
#5301=VERTEX_POINT('',#24711);
#5302=VERTEX_POINT('',#24718);
#5303=VERTEX_POINT('',#24720);
#5304=VERTEX_POINT('',#24727);
#5305=VERTEX_POINT('',#24729);
#5306=VERTEX_POINT('',#24736);
#5307=VERTEX_POINT('',#24738);
#5308=VERTEX_POINT('',#24745);
#5309=VERTEX_POINT('',#24748);
#5310=VERTEX_POINT('',#24750);
#5311=VERTEX_POINT('',#24757);
#5312=VERTEX_POINT('',#24759);
#5313=VERTEX_POINT('',#24768);
#5314=VERTEX_POINT('',#24769);
#5315=VERTEX_POINT('',#24774);
#5316=VERTEX_POINT('',#24797);
#5317=VERTEX_POINT('',#24802);
#5318=VERTEX_POINT('',#24804);
#5319=VERTEX_POINT('',#24809);
#5320=VERTEX_POINT('',#24836);
#5321=VERTEX_POINT('',#24838);
#5322=VERTEX_POINT('',#24862);
#5323=VERTEX_POINT('',#24893);
#5324=VERTEX_POINT('',#24895);
#5325=VERTEX_POINT('',#24897);
#5326=VERTEX_POINT('',#24904);
#5327=VERTEX_POINT('',#24906);
#5328=VERTEX_POINT('',#24913);
#5329=VERTEX_POINT('',#24915);
#5330=VERTEX_POINT('',#24922);
#5331=VERTEX_POINT('',#24924);
#5332=VERTEX_POINT('',#24932);
#5333=VERTEX_POINT('',#24934);
#5334=VERTEX_POINT('',#24941);
#5335=VERTEX_POINT('',#24943);
#5336=VERTEX_POINT('',#24976);
#5337=VERTEX_POINT('',#24978);
#5338=VERTEX_POINT('',#24983);
#5339=VERTEX_POINT('',#24988);
#5340=VERTEX_POINT('',#24990);
#5341=VERTEX_POINT('',#24995);
#5342=VERTEX_POINT('',#25000);
#5343=VERTEX_POINT('',#25002);
#5344=VERTEX_POINT('',#25005);
#5345=VERTEX_POINT('',#25007);
#5346=VERTEX_POINT('',#25012);
#5347=VERTEX_POINT('',#25017);
#5348=VERTEX_POINT('',#25019);
#5349=VERTEX_POINT('',#25024);
#5350=VERTEX_POINT('',#25029);
#5351=VERTEX_POINT('',#25031);
#5352=VERTEX_POINT('',#25036);
#5353=VERTEX_POINT('',#25041);
#5354=VERTEX_POINT('',#25043);
#5355=VERTEX_POINT('',#25048);
#5356=VERTEX_POINT('',#25055);
#5357=VERTEX_POINT('',#25080);
#5358=VERTEX_POINT('',#25081);
#5359=VERTEX_POINT('',#25108);
#5360=VERTEX_POINT('',#25114);
#5361=VERTEX_POINT('',#25164);
#5362=VERTEX_POINT('',#25189);
#5363=VERTEX_POINT('',#25190);
#5364=VERTEX_POINT('',#25217);
#5365=VERTEX_POINT('',#25223);
#5366=VERTEX_POINT('',#25273);
#5367=VERTEX_POINT('',#25275);
#5368=VERTEX_POINT('',#25300);
#5369=VERTEX_POINT('',#25301);
#5370=VERTEX_POINT('',#25328);
#5371=VERTEX_POINT('',#25334);
#5372=VERTEX_POINT('',#25384);
#5373=VERTEX_POINT('',#25409);
#5374=VERTEX_POINT('',#25410);
#5375=VERTEX_POINT('',#25437);
#5376=VERTEX_POINT('',#25443);
#5377=VERTEX_POINT('',#25493);
#5378=VERTEX_POINT('',#25518);
#5379=VERTEX_POINT('',#25523);
#5380=VERTEX_POINT('',#25525);
#5381=VERTEX_POINT('',#25552);
#5382=VERTEX_POINT('',#25578);
#5383=VERTEX_POINT('',#25606);
#5384=VERTEX_POINT('',#25609);
#5385=VERTEX_POINT('',#25611);
#5386=VERTEX_POINT('',#25616);
#5387=VERTEX_POINT('',#25646);
#5388=VERTEX_POINT('',#25670);
#5389=VERTEX_POINT('',#25697);
#5390=VERTEX_POINT('',#25700);
#5391=VERTEX_POINT('',#25704);
#5392=VERTEX_POINT('',#25708);
#5393=VERTEX_POINT('',#25714);
#5394=VERTEX_POINT('',#25716);
#5395=VERTEX_POINT('',#25720);
#5396=VERTEX_POINT('',#25725);
#6816=EDGE_CURVE('',#5289,#5289,#1579,.T.);
#6817=EDGE_CURVE('',#5290,#5290,#1580,.T.);
#6818=EDGE_CURVE('',#5291,#5291,#1581,.T.);
#6819=EDGE_CURVE('',#5292,#5292,#1582,.T.);
#6820=EDGE_CURVE('',#5292,#5290,#3538,.T.);
#6821=EDGE_CURVE('',#5293,#5293,#1583,.T.);
#6822=EDGE_CURVE('',#5293,#5291,#3539,.T.);
#6823=EDGE_CURVE('',#5294,#5294,#1584,.T.);
#6824=EDGE_CURVE('',#5295,#5295,#1585,.T.);
#6825=EDGE_CURVE('',#5296,#5296,#1586,.T.);
#6826=EDGE_CURVE('',#5297,#5297,#1587,.T.);
#6827=EDGE_CURVE('',#5297,#5295,#3540,.T.);
#6828=EDGE_CURVE('',#5298,#5299,#945,.T.);
#6829=EDGE_CURVE('',#5299,#5300,#1588,.T.);
#6830=EDGE_CURVE('',#5300,#5301,#946,.T.);
#6831=EDGE_CURVE('',#5301,#5302,#1589,.T.);
#6832=EDGE_CURVE('',#5302,#5303,#947,.T.);
#6833=EDGE_CURVE('',#5303,#5304,#1590,.T.);
#6834=EDGE_CURVE('',#5304,#5305,#948,.T.);
#6835=EDGE_CURVE('',#5305,#5306,#1591,.T.);
#6836=EDGE_CURVE('',#5306,#5307,#949,.T.);
#6837=EDGE_CURVE('',#5307,#5308,#1592,.T.);
#6838=EDGE_CURVE('',#5308,#5296,#3541,.T.);
#6839=EDGE_CURVE('',#5308,#5309,#1593,.T.);
#6840=EDGE_CURVE('',#5309,#5310,#950,.T.);
#6841=EDGE_CURVE('',#5310,#5311,#1594,.T.);
#6842=EDGE_CURVE('',#5311,#5312,#951,.T.);
#6843=EDGE_CURVE('',#5312,#5298,#1595,.T.);
#6844=EDGE_CURVE('',#5313,#5314,#952,.T.);
#6845=EDGE_CURVE('',#5315,#5313,#953,.T.);
#6846=EDGE_CURVE('',#5316,#5315,#954,.T.);
#6847=EDGE_CURVE('',#5316,#5317,#1596,.T.);
#6848=EDGE_CURVE('',#5318,#5316,#955,.T.);
#6849=EDGE_CURVE('',#5319,#5318,#956,.T.);
#6850=EDGE_CURVE('',#5314,#5319,#957,.T.);
#6851=EDGE_CURVE('',#5320,#5314,#1597,.T.);
#6852=EDGE_CURVE('',#5321,#5298,#958,.T.);
#6853=EDGE_CURVE('',#5322,#5321,#959,.T.);
#6854=EDGE_CURVE('',#5299,#5322,#960,.T.);
#6855=EDGE_CURVE('',#5289,#5323,#3542,.T.);
#6856=EDGE_CURVE('',#5323,#5324,#1598,.T.);
#6857=EDGE_CURVE('',#5324,#5325,#961,.T.);
#6858=EDGE_CURVE('',#5325,#5326,#1599,.T.);
#6859=EDGE_CURVE('',#5326,#5327,#962,.T.);
#6860=EDGE_CURVE('',#5327,#5328,#1600,.T.);
#6861=EDGE_CURVE('',#5328,#5329,#963,.T.);
#6862=EDGE_CURVE('',#5329,#5330,#1601,.T.);
#6863=EDGE_CURVE('',#5330,#5331,#964,.T.);
#6864=EDGE_CURVE('',#5331,#5322,#1602,.T.);
#6865=EDGE_CURVE('',#5321,#5332,#1603,.T.);
#6866=EDGE_CURVE('',#5332,#5333,#965,.T.);
#6867=EDGE_CURVE('',#5333,#5334,#1604,.T.);
#6868=EDGE_CURVE('',#5334,#5335,#966,.T.);
#6869=EDGE_CURVE('',#5335,#5323,#1605,.T.);
#6870=EDGE_CURVE('',#5312,#5332,#967,.T.);
#6871=EDGE_CURVE('',#5315,#5336,#1606,.T.);
#6872=EDGE_CURVE('',#5336,#5337,#968,.T.);
#6873=EDGE_CURVE('',#5337,#5338,#969,.T.);
#6874=EDGE_CURVE('',#5338,#5339,#1607,.T.);
#6875=EDGE_CURVE('',#5339,#5340,#970,.T.);
#6876=EDGE_CURVE('',#5340,#5341,#971,.T.);
#6877=EDGE_CURVE('',#5341,#5342,#1608,.T.);
#6878=EDGE_CURVE('',#5342,#5343,#3543,.T.);
#6879=EDGE_CURVE('',#5343,#5343,#1609,.T.);
#6880=EDGE_CURVE('',#5342,#5344,#1610,.T.);
#6881=EDGE_CURVE('',#5344,#5345,#972,.T.);
#6882=EDGE_CURVE('',#5345,#5346,#973,.T.);
#6883=EDGE_CURVE('',#5346,#5347,#1611,.T.);
#6884=EDGE_CURVE('',#5347,#5348,#974,.T.);
#6885=EDGE_CURVE('',#5348,#5349,#975,.T.);
#6886=EDGE_CURVE('',#5349,#5350,#1612,.T.);
#6887=EDGE_CURVE('',#5350,#5351,#976,.T.);
#6888=EDGE_CURVE('',#5351,#5352,#977,.T.);
#6889=EDGE_CURVE('',#5352,#5353,#1613,.T.);
#6890=EDGE_CURVE('',#5353,#5354,#978,.T.);
#6891=EDGE_CURVE('',#5354,#5355,#979,.T.);
#6892=EDGE_CURVE('',#5355,#5318,#1614,.T.);
#6893=EDGE_CURVE('',#5356,#5313,#1615,.T.);
#6894=EDGE_CURVE('',#5356,#5336,#980,.T.);
#6895=EDGE_CURVE('',#5357,#5358,#981,.T.);
#6896=EDGE_CURVE('',#5338,#5357,#982,.T.);
#6897=EDGE_CURVE('',#5337,#5359,#1616,.T.);
#6898=EDGE_CURVE('',#5358,#5356,#983,.T.);
#6899=EDGE_CURVE('',#5360,#5358,#1617,.T.);
#6900=EDGE_CURVE('',#5333,#5311,#984,.T.);
#6901=EDGE_CURVE('',#5310,#5334,#985,.T.);
#6902=EDGE_CURVE('',#5361,#5357,#1618,.T.);
#6903=EDGE_CURVE('',#5361,#5339,#986,.T.);
#6904=EDGE_CURVE('',#5362,#5363,#987,.T.);
#6905=EDGE_CURVE('',#5341,#5362,#988,.T.);
#6906=EDGE_CURVE('',#5340,#5364,#1619,.T.);
#6907=EDGE_CURVE('',#5363,#5361,#989,.T.);
#6908=EDGE_CURVE('',#5365,#5363,#1620,.T.);
#6909=EDGE_CURVE('',#5335,#5309,#990,.T.);
#6910=EDGE_CURVE('',#5307,#5324,#991,.T.);
#6911=EDGE_CURVE('',#5366,#5362,#1621,.T.);
#6912=EDGE_CURVE('',#5367,#5366,#1622,.T.);
#6913=EDGE_CURVE('',#5367,#5344,#992,.T.);
#6914=EDGE_CURVE('',#5368,#5369,#993,.T.);
#6915=EDGE_CURVE('',#5346,#5368,#994,.T.);
#6916=EDGE_CURVE('',#5345,#5370,#1623,.T.);
#6917=EDGE_CURVE('',#5369,#5367,#995,.T.);
#6918=EDGE_CURVE('',#5371,#5369,#1624,.T.);
#6919=EDGE_CURVE('',#5325,#5306,#996,.T.);
#6920=EDGE_CURVE('',#5305,#5326,#997,.T.);
#6921=EDGE_CURVE('',#5372,#5368,#1625,.T.);
#6922=EDGE_CURVE('',#5372,#5347,#998,.T.);
#6923=EDGE_CURVE('',#5373,#5374,#999,.T.);
#6924=EDGE_CURVE('',#5349,#5373,#1000,.T.);
#6925=EDGE_CURVE('',#5348,#5375,#1626,.T.);
#6926=EDGE_CURVE('',#5374,#5372,#1001,.T.);
#6927=EDGE_CURVE('',#5376,#5374,#1627,.T.);
#6928=EDGE_CURVE('',#5327,#5304,#1002,.T.);
#6929=EDGE_CURVE('',#5303,#5328,#1003,.T.);
#6930=EDGE_CURVE('',#5377,#5373,#1628,.T.);
#6931=EDGE_CURVE('',#5377,#5350,#1004,.T.);
#6932=EDGE_CURVE('',#5378,#5377,#1005,.T.);
#6933=EDGE_CURVE('',#5379,#5378,#1629,.T.);
#6934=EDGE_CURVE('',#5380,#5378,#1006,.T.);
#6935=EDGE_CURVE('',#5352,#5380,#1007,.T.);
#6936=EDGE_CURVE('',#5351,#5381,#1630,.T.);
#6937=EDGE_CURVE('',#5329,#5302,#1008,.T.);
#6938=EDGE_CURVE('',#5294,#5382,#3544,.T.);
#6939=EDGE_CURVE('',#5382,#5382,#1631,.T.);
#6940=EDGE_CURVE('',#5331,#5300,#1009,.T.);
#6941=EDGE_CURVE('',#5383,#5383,#1632,.T.);
#6942=EDGE_CURVE('',#5383,#5366,#3545,.T.);
#6943=EDGE_CURVE('',#5319,#5384,#1633,.T.);
#6944=EDGE_CURVE('',#5384,#5385,#1010,.T.);
#6945=EDGE_CURVE('',#5385,#5386,#1011,.T.);
#6946=EDGE_CURVE('',#5386,#5380,#1634,.T.);
#6947=EDGE_CURVE('',#5355,#5384,#1012,.T.);
#6948=EDGE_CURVE('',#5354,#5387,#1635,.T.);
#6949=EDGE_CURVE('',#5386,#5353,#1013,.T.);
#6950=EDGE_CURVE('',#5388,#5385,#1636,.T.);
#6951=EDGE_CURVE('',#5301,#5330,#1014,.T.);
#6952=EDGE_CURVE('',#5389,#5389,#1637,.T.);
#6953=EDGE_CURVE('',#5390,#5390,#1638,.T.);
#6954=EDGE_CURVE('',#5390,#5389,#3546,.T.);
#6955=EDGE_CURVE('',#5391,#5391,#1639,.T.);
#6956=EDGE_CURVE('',#5391,#5390,#3547,.T.);
#6957=EDGE_CURVE('',#5392,#5392,#1640,.T.);
#6958=EDGE_CURVE('',#5392,#5391,#3548,.T.);
#6959=EDGE_CURVE('',#5393,#5393,#1641,.T.);
#6960=EDGE_CURVE('',#5393,#5394,#3549,.T.);
#6961=EDGE_CURVE('',#5394,#5394,#1642,.T.);
#6962=EDGE_CURVE('',#5394,#5395,#3550,.T.);
#6963=EDGE_CURVE('',#5395,#5395,#1643,.T.);
#6964=EDGE_CURVE('',#5396,#5396,#1644,.T.);
#6965=EDGE_CURVE('',#5396,#5393,#3551,.T.);
#9609=ORIENTED_EDGE('',*,*,#6816,.F.);
#9610=ORIENTED_EDGE('',*,*,#6817,.T.);
#9611=ORIENTED_EDGE('',*,*,#6818,.F.);
#9612=ORIENTED_EDGE('',*,*,#6819,.F.);
#9613=ORIENTED_EDGE('',*,*,#6819,.T.);
#9614=ORIENTED_EDGE('',*,*,#6820,.T.);
#9615=ORIENTED_EDGE('',*,*,#6817,.F.);
#9616=ORIENTED_EDGE('',*,*,#6820,.F.);
#9617=ORIENTED_EDGE('',*,*,#6821,.T.);
#9618=ORIENTED_EDGE('',*,*,#6822,.T.);
#9619=ORIENTED_EDGE('',*,*,#6818,.T.);
#9620=ORIENTED_EDGE('',*,*,#6822,.F.);
#9621=ORIENTED_EDGE('',*,*,#6823,.F.);
#9622=ORIENTED_EDGE('',*,*,#6824,.T.);
#9623=ORIENTED_EDGE('',*,*,#6825,.F.);
#9624=ORIENTED_EDGE('',*,*,#6826,.F.);
#9625=ORIENTED_EDGE('',*,*,#6826,.T.);
#9626=ORIENTED_EDGE('',*,*,#6827,.T.);
#9627=ORIENTED_EDGE('',*,*,#6824,.F.);
#9628=ORIENTED_EDGE('',*,*,#6827,.F.);
#9629=ORIENTED_EDGE('',*,*,#6828,.T.);
#9630=ORIENTED_EDGE('',*,*,#6829,.T.);
#9631=ORIENTED_EDGE('',*,*,#6830,.T.);
#9632=ORIENTED_EDGE('',*,*,#6831,.T.);
#9633=ORIENTED_EDGE('',*,*,#6832,.T.);
#9634=ORIENTED_EDGE('',*,*,#6833,.T.);
#9635=ORIENTED_EDGE('',*,*,#6834,.T.);
#9636=ORIENTED_EDGE('',*,*,#6835,.T.);
#9637=ORIENTED_EDGE('',*,*,#6836,.T.);
#9638=ORIENTED_EDGE('',*,*,#6837,.T.);
#9639=ORIENTED_EDGE('',*,*,#6838,.T.);
#9640=ORIENTED_EDGE('',*,*,#6825,.T.);
#9641=ORIENTED_EDGE('',*,*,#6838,.F.);
#9642=ORIENTED_EDGE('',*,*,#6839,.T.);
#9643=ORIENTED_EDGE('',*,*,#6840,.T.);
#9644=ORIENTED_EDGE('',*,*,#6841,.T.);
#9645=ORIENTED_EDGE('',*,*,#6842,.T.);
#9646=ORIENTED_EDGE('',*,*,#6843,.T.);
#9647=ORIENTED_EDGE('',*,*,#6844,.F.);
#9648=ORIENTED_EDGE('',*,*,#6845,.F.);
#9649=ORIENTED_EDGE('',*,*,#6846,.F.);
#9650=ORIENTED_EDGE('',*,*,#6847,.T.);
#9651=ORIENTED_EDGE('',*,*,#6847,.F.);
#9652=ORIENTED_EDGE('',*,*,#6848,.F.);
#9653=ORIENTED_EDGE('',*,*,#6849,.F.);
#9654=ORIENTED_EDGE('',*,*,#6850,.F.);
#9655=ORIENTED_EDGE('',*,*,#6851,.F.);
#9656=ORIENTED_EDGE('',*,*,#6851,.T.);
#9657=ORIENTED_EDGE('',*,*,#6828,.F.);
#9658=ORIENTED_EDGE('',*,*,#6852,.F.);
#9659=ORIENTED_EDGE('',*,*,#6853,.F.);
#9660=ORIENTED_EDGE('',*,*,#6854,.F.);
#9661=ORIENTED_EDGE('',*,*,#6816,.T.);
#9662=ORIENTED_EDGE('',*,*,#6855,.T.);
#9663=ORIENTED_EDGE('',*,*,#6856,.T.);
#9664=ORIENTED_EDGE('',*,*,#6857,.T.);
#9665=ORIENTED_EDGE('',*,*,#6858,.T.);
#9666=ORIENTED_EDGE('',*,*,#6859,.T.);
#9667=ORIENTED_EDGE('',*,*,#6860,.T.);
#9668=ORIENTED_EDGE('',*,*,#6861,.T.);
#9669=ORIENTED_EDGE('',*,*,#6862,.T.);
#9670=ORIENTED_EDGE('',*,*,#6863,.T.);
#9671=ORIENTED_EDGE('',*,*,#6864,.T.);
#9672=ORIENTED_EDGE('',*,*,#6853,.T.);
#9673=ORIENTED_EDGE('',*,*,#6865,.T.);
#9674=ORIENTED_EDGE('',*,*,#6866,.T.);
#9675=ORIENTED_EDGE('',*,*,#6867,.T.);
#9676=ORIENTED_EDGE('',*,*,#6868,.T.);
#9677=ORIENTED_EDGE('',*,*,#6869,.T.);
#9678=ORIENTED_EDGE('',*,*,#6855,.F.);
#9679=ORIENTED_EDGE('',*,*,#6852,.T.);
#9680=ORIENTED_EDGE('',*,*,#6843,.F.);
#9681=ORIENTED_EDGE('',*,*,#6870,.T.);
#9682=ORIENTED_EDGE('',*,*,#6865,.F.);
#9683=ORIENTED_EDGE('',*,*,#6848,.T.);
#9684=ORIENTED_EDGE('',*,*,#6846,.T.);
#9685=ORIENTED_EDGE('',*,*,#6871,.T.);
#9686=ORIENTED_EDGE('',*,*,#6872,.T.);
#9687=ORIENTED_EDGE('',*,*,#6873,.T.);
#9688=ORIENTED_EDGE('',*,*,#6874,.T.);
#9689=ORIENTED_EDGE('',*,*,#6875,.T.);
#9690=ORIENTED_EDGE('',*,*,#6876,.T.);
#9691=ORIENTED_EDGE('',*,*,#6877,.T.);
#9692=ORIENTED_EDGE('',*,*,#6878,.T.);
#9693=ORIENTED_EDGE('',*,*,#6879,.T.);
#9694=ORIENTED_EDGE('',*,*,#6878,.F.);
#9695=ORIENTED_EDGE('',*,*,#6880,.T.);
#9696=ORIENTED_EDGE('',*,*,#6881,.T.);
#9697=ORIENTED_EDGE('',*,*,#6882,.T.);
#9698=ORIENTED_EDGE('',*,*,#6883,.T.);
#9699=ORIENTED_EDGE('',*,*,#6884,.T.);
#9700=ORIENTED_EDGE('',*,*,#6885,.T.);
#9701=ORIENTED_EDGE('',*,*,#6886,.T.);
#9702=ORIENTED_EDGE('',*,*,#6887,.T.);
#9703=ORIENTED_EDGE('',*,*,#6888,.T.);
#9704=ORIENTED_EDGE('',*,*,#6889,.T.);
#9705=ORIENTED_EDGE('',*,*,#6890,.T.);
#9706=ORIENTED_EDGE('',*,*,#6891,.T.);
#9707=ORIENTED_EDGE('',*,*,#6892,.T.);
#9708=ORIENTED_EDGE('',*,*,#6845,.T.);
#9709=ORIENTED_EDGE('',*,*,#6893,.F.);
#9710=ORIENTED_EDGE('',*,*,#6894,.T.);
#9711=ORIENTED_EDGE('',*,*,#6871,.F.);
#9712=ORIENTED_EDGE('',*,*,#6895,.F.);
#9713=ORIENTED_EDGE('',*,*,#6896,.F.);
#9714=ORIENTED_EDGE('',*,*,#6873,.F.);
#9715=ORIENTED_EDGE('',*,*,#6897,.T.);
#9716=ORIENTED_EDGE('',*,*,#6897,.F.);
#9717=ORIENTED_EDGE('',*,*,#6872,.F.);
#9718=ORIENTED_EDGE('',*,*,#6894,.F.);
#9719=ORIENTED_EDGE('',*,*,#6898,.F.);
#9720=ORIENTED_EDGE('',*,*,#6899,.F.);
#9721=ORIENTED_EDGE('',*,*,#6899,.T.);
#9722=ORIENTED_EDGE('',*,*,#6842,.F.);
#9723=ORIENTED_EDGE('',*,*,#6900,.F.);
#9724=ORIENTED_EDGE('',*,*,#6866,.F.);
#9725=ORIENTED_EDGE('',*,*,#6870,.F.);
#9726=ORIENTED_EDGE('',*,*,#6900,.T.);
#9727=ORIENTED_EDGE('',*,*,#6841,.F.);
#9728=ORIENTED_EDGE('',*,*,#6901,.T.);
#9729=ORIENTED_EDGE('',*,*,#6867,.F.);
#9730=ORIENTED_EDGE('',*,*,#6896,.T.);
#9731=ORIENTED_EDGE('',*,*,#6902,.F.);
#9732=ORIENTED_EDGE('',*,*,#6903,.T.);
#9733=ORIENTED_EDGE('',*,*,#6874,.F.);
#9734=ORIENTED_EDGE('',*,*,#6904,.F.);
#9735=ORIENTED_EDGE('',*,*,#6905,.F.);
#9736=ORIENTED_EDGE('',*,*,#6876,.F.);
#9737=ORIENTED_EDGE('',*,*,#6906,.T.);
#9738=ORIENTED_EDGE('',*,*,#6906,.F.);
#9739=ORIENTED_EDGE('',*,*,#6875,.F.);
#9740=ORIENTED_EDGE('',*,*,#6903,.F.);
#9741=ORIENTED_EDGE('',*,*,#6907,.F.);
#9742=ORIENTED_EDGE('',*,*,#6908,.F.);
#9743=ORIENTED_EDGE('',*,*,#6908,.T.);
#9744=ORIENTED_EDGE('',*,*,#6840,.F.);
#9745=ORIENTED_EDGE('',*,*,#6909,.F.);
#9746=ORIENTED_EDGE('',*,*,#6868,.F.);
#9747=ORIENTED_EDGE('',*,*,#6901,.F.);
#9748=ORIENTED_EDGE('',*,*,#6909,.T.);
#9749=ORIENTED_EDGE('',*,*,#6839,.F.);
#9750=ORIENTED_EDGE('',*,*,#6837,.F.);
#9751=ORIENTED_EDGE('',*,*,#6910,.T.);
#9752=ORIENTED_EDGE('',*,*,#6856,.F.);
#9753=ORIENTED_EDGE('',*,*,#6869,.F.);
#9754=ORIENTED_EDGE('',*,*,#6905,.T.);
#9755=ORIENTED_EDGE('',*,*,#6911,.F.);
#9756=ORIENTED_EDGE('',*,*,#6912,.F.);
#9757=ORIENTED_EDGE('',*,*,#6913,.T.);
#9758=ORIENTED_EDGE('',*,*,#6880,.F.);
#9759=ORIENTED_EDGE('',*,*,#6877,.F.);
#9760=ORIENTED_EDGE('',*,*,#6914,.F.);
#9761=ORIENTED_EDGE('',*,*,#6915,.F.);
#9762=ORIENTED_EDGE('',*,*,#6882,.F.);
#9763=ORIENTED_EDGE('',*,*,#6916,.T.);
#9764=ORIENTED_EDGE('',*,*,#6916,.F.);
#9765=ORIENTED_EDGE('',*,*,#6881,.F.);
#9766=ORIENTED_EDGE('',*,*,#6913,.F.);
#9767=ORIENTED_EDGE('',*,*,#6917,.F.);
#9768=ORIENTED_EDGE('',*,*,#6918,.F.);
#9769=ORIENTED_EDGE('',*,*,#6918,.T.);
#9770=ORIENTED_EDGE('',*,*,#6836,.F.);
#9771=ORIENTED_EDGE('',*,*,#6919,.F.);
#9772=ORIENTED_EDGE('',*,*,#6857,.F.);
#9773=ORIENTED_EDGE('',*,*,#6910,.F.);
#9774=ORIENTED_EDGE('',*,*,#6919,.T.);
#9775=ORIENTED_EDGE('',*,*,#6835,.F.);
#9776=ORIENTED_EDGE('',*,*,#6920,.T.);
#9777=ORIENTED_EDGE('',*,*,#6858,.F.);
#9778=ORIENTED_EDGE('',*,*,#6915,.T.);
#9779=ORIENTED_EDGE('',*,*,#6921,.F.);
#9780=ORIENTED_EDGE('',*,*,#6922,.T.);
#9781=ORIENTED_EDGE('',*,*,#6883,.F.);
#9782=ORIENTED_EDGE('',*,*,#6923,.F.);
#9783=ORIENTED_EDGE('',*,*,#6924,.F.);
#9784=ORIENTED_EDGE('',*,*,#6885,.F.);
#9785=ORIENTED_EDGE('',*,*,#6925,.T.);
#9786=ORIENTED_EDGE('',*,*,#6925,.F.);
#9787=ORIENTED_EDGE('',*,*,#6884,.F.);
#9788=ORIENTED_EDGE('',*,*,#6922,.F.);
#9789=ORIENTED_EDGE('',*,*,#6926,.F.);
#9790=ORIENTED_EDGE('',*,*,#6927,.F.);
#9791=ORIENTED_EDGE('',*,*,#6927,.T.);
#9792=ORIENTED_EDGE('',*,*,#6834,.F.);
#9793=ORIENTED_EDGE('',*,*,#6928,.F.);
#9794=ORIENTED_EDGE('',*,*,#6859,.F.);
#9795=ORIENTED_EDGE('',*,*,#6920,.F.);
#9796=ORIENTED_EDGE('',*,*,#6928,.T.);
#9797=ORIENTED_EDGE('',*,*,#6833,.F.);
#9798=ORIENTED_EDGE('',*,*,#6929,.T.);
#9799=ORIENTED_EDGE('',*,*,#6860,.F.);
#9800=ORIENTED_EDGE('',*,*,#6924,.T.);
#9801=ORIENTED_EDGE('',*,*,#6930,.F.);
#9802=ORIENTED_EDGE('',*,*,#6931,.T.);
#9803=ORIENTED_EDGE('',*,*,#6886,.F.);
#9804=ORIENTED_EDGE('',*,*,#6887,.F.);
#9805=ORIENTED_EDGE('',*,*,#6931,.F.);
#9806=ORIENTED_EDGE('',*,*,#6932,.F.);
#9807=ORIENTED_EDGE('',*,*,#6933,.F.);
#9808=ORIENTED_EDGE('',*,*,#6933,.T.);
#9809=ORIENTED_EDGE('',*,*,#6934,.F.);
#9810=ORIENTED_EDGE('',*,*,#6935,.F.);
#9811=ORIENTED_EDGE('',*,*,#6888,.F.);
#9812=ORIENTED_EDGE('',*,*,#6936,.T.);
#9813=ORIENTED_EDGE('',*,*,#6936,.F.);
#9814=ORIENTED_EDGE('',*,*,#6861,.F.);
#9815=ORIENTED_EDGE('',*,*,#6929,.F.);
#9816=ORIENTED_EDGE('',*,*,#6832,.F.);
#9817=ORIENTED_EDGE('',*,*,#6937,.F.);
#9818=ORIENTED_EDGE('',*,*,#6823,.T.);
#9819=ORIENTED_EDGE('',*,*,#6938,.T.);
#9820=ORIENTED_EDGE('',*,*,#6939,.F.);
#9821=ORIENTED_EDGE('',*,*,#6938,.F.);
#9822=ORIENTED_EDGE('',*,*,#6854,.T.);
#9823=ORIENTED_EDGE('',*,*,#6864,.F.);
#9824=ORIENTED_EDGE('',*,*,#6940,.T.);
#9825=ORIENTED_EDGE('',*,*,#6829,.F.);
#9826=ORIENTED_EDGE('',*,*,#6941,.F.);
#9827=ORIENTED_EDGE('',*,*,#6942,.T.);
#9828=ORIENTED_EDGE('',*,*,#6911,.T.);
#9829=ORIENTED_EDGE('',*,*,#6904,.T.);
#9830=ORIENTED_EDGE('',*,*,#6907,.T.);
#9831=ORIENTED_EDGE('',*,*,#6902,.T.);
#9832=ORIENTED_EDGE('',*,*,#6895,.T.);
#9833=ORIENTED_EDGE('',*,*,#6898,.T.);
#9834=ORIENTED_EDGE('',*,*,#6893,.T.);
#9835=ORIENTED_EDGE('',*,*,#6844,.T.);
#9836=ORIENTED_EDGE('',*,*,#6850,.T.);
#9837=ORIENTED_EDGE('',*,*,#6943,.T.);
#9838=ORIENTED_EDGE('',*,*,#6944,.T.);
#9839=ORIENTED_EDGE('',*,*,#6945,.T.);
#9840=ORIENTED_EDGE('',*,*,#6946,.T.);
#9841=ORIENTED_EDGE('',*,*,#6934,.T.);
#9842=ORIENTED_EDGE('',*,*,#6932,.T.);
#9843=ORIENTED_EDGE('',*,*,#6930,.T.);
#9844=ORIENTED_EDGE('',*,*,#6923,.T.);
#9845=ORIENTED_EDGE('',*,*,#6926,.T.);
#9846=ORIENTED_EDGE('',*,*,#6921,.T.);
#9847=ORIENTED_EDGE('',*,*,#6914,.T.);
#9848=ORIENTED_EDGE('',*,*,#6917,.T.);
#9849=ORIENTED_EDGE('',*,*,#6912,.T.);
#9850=ORIENTED_EDGE('',*,*,#6942,.F.);
#9851=ORIENTED_EDGE('',*,*,#6849,.T.);
#9852=ORIENTED_EDGE('',*,*,#6892,.F.);
#9853=ORIENTED_EDGE('',*,*,#6947,.T.);
#9854=ORIENTED_EDGE('',*,*,#6943,.F.);
#9855=ORIENTED_EDGE('',*,*,#6947,.F.);
#9856=ORIENTED_EDGE('',*,*,#6891,.F.);
#9857=ORIENTED_EDGE('',*,*,#6948,.T.);
#9858=ORIENTED_EDGE('',*,*,#6948,.F.);
#9859=ORIENTED_EDGE('',*,*,#6890,.F.);
#9860=ORIENTED_EDGE('',*,*,#6949,.F.);
#9861=ORIENTED_EDGE('',*,*,#6945,.F.);
#9862=ORIENTED_EDGE('',*,*,#6950,.F.);
#9863=ORIENTED_EDGE('',*,*,#6950,.T.);
#9864=ORIENTED_EDGE('',*,*,#6944,.F.);
#9865=ORIENTED_EDGE('',*,*,#6940,.F.);
#9866=ORIENTED_EDGE('',*,*,#6863,.F.);
#9867=ORIENTED_EDGE('',*,*,#6951,.F.);
#9868=ORIENTED_EDGE('',*,*,#6830,.F.);
#9869=ORIENTED_EDGE('',*,*,#6937,.T.);
#9870=ORIENTED_EDGE('',*,*,#6831,.F.);
#9871=ORIENTED_EDGE('',*,*,#6951,.T.);
#9872=ORIENTED_EDGE('',*,*,#6862,.F.);
#9873=ORIENTED_EDGE('',*,*,#6952,.F.);
#9874=ORIENTED_EDGE('',*,*,#6939,.T.);
#9875=ORIENTED_EDGE('',*,*,#6953,.F.);
#9876=ORIENTED_EDGE('',*,*,#6954,.T.);
#9877=ORIENTED_EDGE('',*,*,#6952,.T.);
#9878=ORIENTED_EDGE('',*,*,#6954,.F.);
#9879=ORIENTED_EDGE('',*,*,#6955,.F.);
#9880=ORIENTED_EDGE('',*,*,#6956,.T.);
#9881=ORIENTED_EDGE('',*,*,#6953,.T.);
#9882=ORIENTED_EDGE('',*,*,#6956,.F.);
#9883=ORIENTED_EDGE('',*,*,#6957,.F.);
#9884=ORIENTED_EDGE('',*,*,#6958,.T.);
#9885=ORIENTED_EDGE('',*,*,#6955,.T.);
#9886=ORIENTED_EDGE('',*,*,#6958,.F.);
#9887=ORIENTED_EDGE('',*,*,#6957,.T.);
#9888=ORIENTED_EDGE('',*,*,#6821,.F.);
#9889=ORIENTED_EDGE('',*,*,#6935,.T.);
#9890=ORIENTED_EDGE('',*,*,#6946,.F.);
#9891=ORIENTED_EDGE('',*,*,#6949,.T.);
#9892=ORIENTED_EDGE('',*,*,#6889,.F.);
#9893=ORIENTED_EDGE('',*,*,#6959,.T.);
#9894=ORIENTED_EDGE('',*,*,#6960,.T.);
#9895=ORIENTED_EDGE('',*,*,#6961,.F.);
#9896=ORIENTED_EDGE('',*,*,#6960,.F.);
#9897=ORIENTED_EDGE('',*,*,#6961,.T.);
#9898=ORIENTED_EDGE('',*,*,#6962,.T.);
#9899=ORIENTED_EDGE('',*,*,#6963,.F.);
#9900=ORIENTED_EDGE('',*,*,#6962,.F.);
#9901=ORIENTED_EDGE('',*,*,#6879,.F.);
#9902=ORIENTED_EDGE('',*,*,#6963,.T.);
#9903=ORIENTED_EDGE('',*,*,#6941,.T.);
#9904=ORIENTED_EDGE('',*,*,#6964,.F.);
#9905=ORIENTED_EDGE('',*,*,#6964,.T.);
#9906=ORIENTED_EDGE('',*,*,#6965,.T.);
#9907=ORIENTED_EDGE('',*,*,#6959,.F.);
#9908=ORIENTED_EDGE('',*,*,#6965,.F.);
#11573=PLANE('',#12987);
#11574=PLANE('',#12990);
#11575=PLANE('',#12996);
#11576=PLANE('',#12999);
#11577=PLANE('',#13077);
#11578=PLANE('',#13085);
#11579=PLANE('',#13092);
#11580=PLANE('',#13093);
#12124=ADVANCED_FACE('',(#2157,#1375),#11573,.T.);
#12125=ADVANCED_FACE('',(#2158,#1376),#11574,.T.);
#12126=ADVANCED_FACE('',(#2159),#277,.F.);
#12127=ADVANCED_FACE('',(#2160),#278,.F.);
#12128=ADVANCED_FACE('',(#2161,#1377),#11575,.T.);
#12129=ADVANCED_FACE('',(#2162,#1378),#11576,.T.);
#12130=ADVANCED_FACE('',(#2163),#279,.F.);
#12131=ADVANCED_FACE('',(#2164),#280,.F.);
#12132=ADVANCED_FACE('',(#2165,#1379),#176,.T.);
#12133=ADVANCED_FACE('',(#2166),#281,.F.);
#12134=ADVANCED_FACE('',(#2167),#231,.F.);
#12135=ADVANCED_FACE('',(#2168),#282,.T.);
#12136=ADVANCED_FACE('',(#2169),#232,.F.);
#12137=ADVANCED_FACE('',(#2170,#1380),#177,.T.);
#12138=ADVANCED_FACE('',(#2171),#233,.F.);
#12139=ADVANCED_FACE('',(#2172),#234,.F.);
#12140=ADVANCED_FACE('',(#2173,#1381),#178,.T.);
#12141=ADVANCED_FACE('',(#2174),#235,.F.);
#12142=ADVANCED_FACE('',(#2175),#236,.F.);
#12143=ADVANCED_FACE('',(#2176,#1382),#179,.T.);
#12144=ADVANCED_FACE('',(#2177),#237,.F.);
#12145=ADVANCED_FACE('',(#2178),#238,.F.);
#12146=ADVANCED_FACE('',(#2179,#1383),#180,.T.);
#12147=ADVANCED_FACE('',(#2180),#239,.F.);
#12148=ADVANCED_FACE('',(#2181),#240,.F.);
#12149=ADVANCED_FACE('',(#2182,#1384),#181,.T.);
#12150=ADVANCED_FACE('',(#2183),#283,.F.);
#12151=ADVANCED_FACE('',(#2184),#241,.F.);
#12152=ADVANCED_FACE('',(#2185),#284,.T.);
#12153=ADVANCED_FACE('',(#2186),#242,.F.);
#12154=ADVANCED_FACE('',(#2187,#1385),#182,.T.);
#12155=ADVANCED_FACE('',(#2188),#243,.F.);
#12156=ADVANCED_FACE('',(#2189,#1386),#11577,.T.);
#12157=ADVANCED_FACE('',(#2190),#431,.T.);
#12158=ADVANCED_FACE('',(#2191),#285,.T.);
#12159=ADVANCED_FACE('',(#2192),#432,.T.);
#12160=ADVANCED_FACE('',(#2193,#1387),#11578,.T.);
#12161=ADVANCED_FACE('',(#2194),#244,.F.);
#12162=ADVANCED_FACE('',(#2195),#286,.F.);
#12163=ADVANCED_FACE('',(#2196),#433,.F.);
#12164=ADVANCED_FACE('',(#2197,#1388),#11579,.T.);
#12165=ADVANCED_FACE('',(#2198,#1389),#11580,.T.);
#12166=ADVANCED_FACE('',(#2199),#434,.F.);
#12484=CLOSED_SHELL('',(#12124,#12125,#12126,#12127,#12128,#12129,#12130,
#12131,#12132,#12133,#12134,#12135,#12136,#12137,#12138,#12139,#12140,#12141,
#12142,#12143,#12144,#12145,#12146,#12147,#12148,#12149,#12150,#12151,#12152,
#12153,#12154,#12155,#12156,#12157,#12158,#12159,#12160,#12161,#12162,#12163,
#12164,#12165,#12166));
#12986=AXIS2_PLACEMENT_3D('',#24671,#14632,#14633);
#12987=AXIS2_PLACEMENT_3D('',#24672,#14634,#14635);
#12988=AXIS2_PLACEMENT_3D('',#24674,#14636,#14637);
#12989=AXIS2_PLACEMENT_3D('',#24676,#14638,#14639);
#12990=AXIS2_PLACEMENT_3D('',#24677,#14640,#14641);
#12991=AXIS2_PLACEMENT_3D('',#24679,#14642,#14643);
#12992=AXIS2_PLACEMENT_3D('',#24681,#14644,#14645);
#12993=AXIS2_PLACEMENT_3D('',#24682,#14646,#14647);
#12994=AXIS2_PLACEMENT_3D('',#24684,#14649,#14650);
#12995=AXIS2_PLACEMENT_3D('',#24686,#14651,#14652);
#12996=AXIS2_PLACEMENT_3D('',#24688,#14654,#14655);
#12997=AXIS2_PLACEMENT_3D('',#24690,#14656,#14657);
#12998=AXIS2_PLACEMENT_3D('',#24692,#14658,#14659);
#12999=AXIS2_PLACEMENT_3D('',#24693,#14660,#14661);
#13000=AXIS2_PLACEMENT_3D('',#24695,#14662,#14663);
#13001=AXIS2_PLACEMENT_3D('',#24697,#14664,#14665);
#13002=AXIS2_PLACEMENT_3D('',#24698,#14666,#14667);
#13003=AXIS2_PLACEMENT_3D('',#24700,#14669,#14670);
#13004=AXIS2_PLACEMENT_3D('',#24710,#14671,#14672);
#13005=AXIS2_PLACEMENT_3D('',#24719,#14673,#14674);
#13006=AXIS2_PLACEMENT_3D('',#24728,#14675,#14676);
#13007=AXIS2_PLACEMENT_3D('',#24737,#14677,#14678);
#13008=AXIS2_PLACEMENT_3D('',#24746,#14679,#14680);
#13009=AXIS2_PLACEMENT_3D('',#24749,#14682,#14683);
#13010=AXIS2_PLACEMENT_3D('',#24758,#14684,#14685);
#13011=AXIS2_PLACEMENT_3D('',#24766,#14686,#14687);
#13012=AXIS2_PLACEMENT_3D('',#24767,#14688,#14689);
#13013=AXIS2_PLACEMENT_3D('',#24803,#14690,#14691);
#13014=AXIS2_PLACEMENT_3D('',#24837,#14692,#14693);
#13015=AXIS2_PLACEMENT_3D('',#24892,#14694,#14695);
#13016=AXIS2_PLACEMENT_3D('',#24896,#14697,#14698);
#13017=AXIS2_PLACEMENT_3D('',#24905,#14699,#14700);
#13018=AXIS2_PLACEMENT_3D('',#24914,#14701,#14702);
#13019=AXIS2_PLACEMENT_3D('',#24923,#14703,#14704);
#13020=AXIS2_PLACEMENT_3D('',#24931,#14705,#14706);
#13021=AXIS2_PLACEMENT_3D('',#24933,#14707,#14708);
#13022=AXIS2_PLACEMENT_3D('',#24942,#14709,#14710);
#13023=AXIS2_PLACEMENT_3D('',#24950,#14711,#14712);
#13024=AXIS2_PLACEMENT_3D('',#24951,#14713,#14714);
#13025=AXIS2_PLACEMENT_3D('',#24975,#14715,#14716);
#13026=AXIS2_PLACEMENT_3D('',#24977,#14717,#14718);
#13027=AXIS2_PLACEMENT_3D('',#24989,#14719,#14720);
#13028=AXIS2_PLACEMENT_3D('',#25001,#14721,#14722);
#13029=AXIS2_PLACEMENT_3D('',#25004,#14724,#14725);
#13030=AXIS2_PLACEMENT_3D('',#25006,#14726,#14727);
#13031=AXIS2_PLACEMENT_3D('',#25018,#14728,#14729);
#13032=AXIS2_PLACEMENT_3D('',#25030,#14730,#14731);
#13033=AXIS2_PLACEMENT_3D('',#25042,#14732,#14733);
#13034=AXIS2_PLACEMENT_3D('',#25053,#14734,#14735);
#13035=AXIS2_PLACEMENT_3D('',#25054,#14736,#14737);
#13036=AXIS2_PLACEMENT_3D('',#25056,#14738,#14739);
#13037=AXIS2_PLACEMENT_3D('',#25079,#14740,#14741);
#13038=AXIS2_PLACEMENT_3D('',#25109,#14742,#14743);
#13039=AXIS2_PLACEMENT_3D('',#25115,#14744,#14745);
#13040=AXIS2_PLACEMENT_3D('',#25139,#14746,#14747);
#13041=AXIS2_PLACEMENT_3D('',#25163,#14748,#14749);
#13042=AXIS2_PLACEMENT_3D('',#25165,#14750,#14751);
#13043=AXIS2_PLACEMENT_3D('',#25188,#14752,#14753);
#13044=AXIS2_PLACEMENT_3D('',#25218,#14754,#14755);
#13045=AXIS2_PLACEMENT_3D('',#25224,#14756,#14757);
#13046=AXIS2_PLACEMENT_3D('',#25248,#14758,#14759);
#13047=AXIS2_PLACEMENT_3D('',#25272,#14760,#14761);
#13048=AXIS2_PLACEMENT_3D('',#25274,#14762,#14763);
#13049=AXIS2_PLACEMENT_3D('',#25276,#14764,#14765);
#13050=AXIS2_PLACEMENT_3D('',#25299,#14766,#14767);
#13051=AXIS2_PLACEMENT_3D('',#25329,#14768,#14769);
#13052=AXIS2_PLACEMENT_3D('',#25335,#14770,#14771);
#13053=AXIS2_PLACEMENT_3D('',#25359,#14772,#14773);
#13054=AXIS2_PLACEMENT_3D('',#25383,#14774,#14775);
#13055=AXIS2_PLACEMENT_3D('',#25385,#14776,#14777);
#13056=AXIS2_PLACEMENT_3D('',#25408,#14778,#14779);
#13057=AXIS2_PLACEMENT_3D('',#25438,#14780,#14781);
#13058=AXIS2_PLACEMENT_3D('',#25444,#14782,#14783);
#13059=AXIS2_PLACEMENT_3D('',#25468,#14784,#14785);
#13060=AXIS2_PLACEMENT_3D('',#25492,#14786,#14787);
#13061=AXIS2_PLACEMENT_3D('',#25494,#14788,#14789);
#13062=AXIS2_PLACEMENT_3D('',#25517,#14790,#14791);
#13063=AXIS2_PLACEMENT_3D('',#25524,#14792,#14793);
#13064=AXIS2_PLACEMENT_3D('',#25553,#14794,#14795);
#13065=AXIS2_PLACEMENT_3D('',#25577,#14796,#14797);
#13066=AXIS2_PLACEMENT_3D('',#25580,#14799,#14800);
#13067=AXIS2_PLACEMENT_3D('',#25581,#14801,#14802);
#13068=AXIS2_PLACEMENT_3D('',#25605,#14803,#14804);
#13069=AXIS2_PLACEMENT_3D('',#25607,#14805,#14806);
#13070=AXIS2_PLACEMENT_3D('',#25610,#14808,#14809);
#13071=AXIS2_PLACEMENT_3D('',#25621,#14810,#14811);
#13072=AXIS2_PLACEMENT_3D('',#25622,#14812,#14813);
#13073=AXIS2_PLACEMENT_3D('',#25645,#14814,#14815);
#13074=AXIS2_PLACEMENT_3D('',#25647,#14816,#14817);
#13075=AXIS2_PLACEMENT_3D('',#25671,#14818,#14819);
#13076=AXIS2_PLACEMENT_3D('',#25695,#14820,#14821);
#13077=AXIS2_PLACEMENT_3D('',#25696,#14822,#14823);
#13078=AXIS2_PLACEMENT_3D('',#25698,#14824,#14825);
#13079=AXIS2_PLACEMENT_3D('',#25699,#14826,#14827);
#13080=AXIS2_PLACEMENT_3D('',#25701,#14828,#14829);
#13081=AXIS2_PLACEMENT_3D('',#25703,#14831,#14832);
#13082=AXIS2_PLACEMENT_3D('',#25705,#14833,#14834);
#13083=AXIS2_PLACEMENT_3D('',#25707,#14836,#14837);
#13084=AXIS2_PLACEMENT_3D('',#25709,#14838,#14839);
#13085=AXIS2_PLACEMENT_3D('',#25711,#14841,#14842);
#13086=AXIS2_PLACEMENT_3D('',#25712,#14843,#14844);
#13087=AXIS2_PLACEMENT_3D('',#25713,#14845,#14846);
#13088=AXIS2_PLACEMENT_3D('',#25715,#14847,#14848);
#13089=AXIS2_PLACEMENT_3D('',#25718,#14850,#14851);
#13090=AXIS2_PLACEMENT_3D('',#25719,#14852,#14853);
#13091=AXIS2_PLACEMENT_3D('',#25722,#14855,#14856);
#13092=AXIS2_PLACEMENT_3D('',#25723,#14857,#14858);
#13093=AXIS2_PLACEMENT_3D('',#25724,#14859,#14860);
#13094=AXIS2_PLACEMENT_3D('',#25726,#14861,#14862);
#13095=AXIS2_PLACEMENT_3D('',#25727,#14863,#14864);
#14632=DIRECTION('axis',(0.,0.,1.));
#14633=DIRECTION('refdir',(1.,0.,0.));
#14634=DIRECTION('center_axis',(0.,0.,-1.));
#14635=DIRECTION('ref_axis',(-1.,0.,0.));
#14636=DIRECTION('center_axis',(0.,0.,1.));
#14637=DIRECTION('ref_axis',(1.,0.,0.));
#14638=DIRECTION('center_axis',(0.,0.,1.));
#14639=DIRECTION('ref_axis',(1.,0.,0.));
#14640=DIRECTION('center_axis',(0.,0.,1.));
#14641=DIRECTION('ref_axis',(1.,0.,0.));
#14642=DIRECTION('center_axis',(0.,0.,-1.));
#14643=DIRECTION('ref_axis',(1.,0.,0.));
#14644=DIRECTION('center_axis',(0.,0.,1.));
#14645=DIRECTION('ref_axis',(1.,0.,0.));
#14646=DIRECTION('center_axis',(0.,0.,1.));
#14647=DIRECTION('ref_axis',(1.,0.,0.));
#14648=DIRECTION('',(0.,0.,-1.));
#14649=DIRECTION('center_axis',(0.,0.,1.));
#14650=DIRECTION('ref_axis',(1.,0.,0.));
#14651=DIRECTION('center_axis',(0.,0.,1.));
#14652=DIRECTION('ref_axis',(1.,0.,0.));
#14653=DIRECTION('',(0.,0.,-1.));
#14654=DIRECTION('center_axis',(0.,0.,-1.));
#14655=DIRECTION('ref_axis',(-1.,0.,0.));
#14656=DIRECTION('center_axis',(0.,0.,1.));
#14657=DIRECTION('ref_axis',(1.,0.,0.));
#14658=DIRECTION('center_axis',(0.,0.,1.));
#14659=DIRECTION('ref_axis',(1.,0.,0.));
#14660=DIRECTION('center_axis',(0.,0.,1.));
#14661=DIRECTION('ref_axis',(1.,0.,0.));
#14662=DIRECTION('center_axis',(0.,0.,-1.));
#14663=DIRECTION('ref_axis',(1.,0.,0.));
#14664=DIRECTION('center_axis',(0.,0.,1.));
#14665=DIRECTION('ref_axis',(1.,0.,0.));
#14666=DIRECTION('center_axis',(0.,0.,1.));
#14667=DIRECTION('ref_axis',(1.,0.,0.));
#14668=DIRECTION('',(0.,0.,-1.));
#14669=DIRECTION('center_axis',(0.,0.,1.));
#14670=DIRECTION('ref_axis',(1.,0.,0.));
#14671=DIRECTION('center_axis',(0.,0.,1.));
#14672=DIRECTION('ref_axis',(1.,0.,0.));
#14673=DIRECTION('center_axis',(0.,0.,1.));
#14674=DIRECTION('ref_axis',(1.,0.,0.));
#14675=DIRECTION('center_axis',(0.,0.,1.));
#14676=DIRECTION('ref_axis',(1.,0.,0.));
#14677=DIRECTION('center_axis',(0.,0.,1.));
#14678=DIRECTION('ref_axis',(1.,0.,0.));
#14679=DIRECTION('center_axis',(0.,0.,1.));
#14680=DIRECTION('ref_axis',(1.,0.,0.));
#14681=DIRECTION('',(0.,0.,-1.));
#14682=DIRECTION('center_axis',(0.,0.,1.));
#14683=DIRECTION('ref_axis',(1.,0.,0.));
#14684=DIRECTION('center_axis',(0.,0.,1.));
#14685=DIRECTION('ref_axis',(1.,0.,0.));
#14686=DIRECTION('center_axis',(0.,0.,1.));
#14687=DIRECTION('ref_axis',(1.,0.,0.));
#14688=DIRECTION('center_axis',(0.,0.,1.));
#14689=DIRECTION('ref_axis',(0.623489801858733,-0.78183148246803,0.));
#14690=DIRECTION('center_axis',(-0.78183148246803,-0.623489801858733,0.));
#14691=DIRECTION('ref_axis',(-0.623489801858733,0.78183148246803,0.));
#14692=DIRECTION('center_axis',(-0.78183148246803,-0.623489801858733,0.));
#14693=DIRECTION('ref_axis',(-0.623489801858733,0.78183148246803,0.));
#14694=DIRECTION('center_axis',(0.,0.,1.));
#14695=DIRECTION('ref_axis',(1.,0.,0.));
#14696=DIRECTION('',(0.,0.,-1.));
#14697=DIRECTION('center_axis',(0.,0.,-1.));
#14698=DIRECTION('ref_axis',(1.,0.,0.));
#14699=DIRECTION('center_axis',(0.,0.,-1.));
#14700=DIRECTION('ref_axis',(1.,0.,0.));
#14701=DIRECTION('center_axis',(0.,0.,-1.));
#14702=DIRECTION('ref_axis',(1.,0.,0.));
#14703=DIRECTION('center_axis',(0.,0.,-1.));
#14704=DIRECTION('ref_axis',(1.,0.,0.));
#14705=DIRECTION('center_axis',(0.,0.,-1.));
#14706=DIRECTION('ref_axis',(1.,0.,0.));
#14707=DIRECTION('center_axis',(0.,0.,-1.));
#14708=DIRECTION('ref_axis',(1.,0.,0.));
#14709=DIRECTION('center_axis',(0.,0.,-1.));
#14710=DIRECTION('ref_axis',(1.,0.,0.));
#14711=DIRECTION('center_axis',(0.,0.,-1.));
#14712=DIRECTION('ref_axis',(1.,0.,0.));
#14713=DIRECTION('center_axis',(0.,0.,1.));
#14714=DIRECTION('ref_axis',(1.,0.,0.));
#14715=DIRECTION('center_axis',(0.,0.,1.));
#14716=DIRECTION('ref_axis',(1.,0.,0.));
#14717=DIRECTION('center_axis',(0.,0.,-1.));
#14718=DIRECTION('ref_axis',(1.,0.,0.));
#14719=DIRECTION('center_axis',(0.,0.,-1.));
#14720=DIRECTION('ref_axis',(1.,0.,0.));
#14721=DIRECTION('center_axis',(0.,0.,-1.));
#14722=DIRECTION('ref_axis',(1.,0.,0.));
#14723=DIRECTION('',(0.,0.,-1.));
#14724=DIRECTION('center_axis',(0.,0.,1.));
#14725=DIRECTION('ref_axis',(1.,0.,0.));
#14726=DIRECTION('center_axis',(0.,0.,-1.));
#14727=DIRECTION('ref_axis',(1.,0.,0.));
#14728=DIRECTION('center_axis',(0.,0.,-1.));
#14729=DIRECTION('ref_axis',(1.,0.,0.));
#14730=DIRECTION('center_axis',(0.,0.,-1.));
#14731=DIRECTION('ref_axis',(1.,0.,0.));
#14732=DIRECTION('center_axis',(0.,0.,-1.));
#14733=DIRECTION('ref_axis',(1.,0.,0.));
#14734=DIRECTION('center_axis',(0.,0.,-1.));
#14735=DIRECTION('ref_axis',(1.,0.,0.));
#14736=DIRECTION('center_axis',(0.,0.,1.));
#14737=DIRECTION('ref_axis',(1.,0.,0.));
#14738=DIRECTION('center_axis',(0.,0.,1.));
#14739=DIRECTION('ref_axis',(1.,0.,0.));
#14740=DIRECTION('center_axis',(0.,0.,1.));
#14741=DIRECTION('ref_axis',(-0.222520933956315,-0.974927912181824,0.));
#14742=DIRECTION('center_axis',(-0.974927912181824,0.222520933956314,0.));
#14743=DIRECTION('ref_axis',(0.222520933956314,0.974927912181824,0.));
#14744=DIRECTION('center_axis',(-0.974927912181824,0.222520933956314,0.));
#14745=DIRECTION('ref_axis',(0.222520933956314,0.974927912181824,0.));
#14746=DIRECTION('center_axis',(0.,0.,1.));
#14747=DIRECTION('ref_axis',(1.,0.,0.));
#14748=DIRECTION('center_axis',(0.,0.,1.));
#14749=DIRECTION('ref_axis',(1.,0.,0.));
#14750=DIRECTION('center_axis',(0.,0.,1.));
#14751=DIRECTION('ref_axis',(1.,0.,0.));
#14752=DIRECTION('center_axis',(0.,0.,1.));
#14753=DIRECTION('ref_axis',(-0.900968867902419,-0.433883739117558,0.));
#14754=DIRECTION('center_axis',(-0.433883739117558,0.900968867902419,0.));
#14755=DIRECTION('ref_axis',(0.900968867902419,0.433883739117558,0.));
#14756=DIRECTION('center_axis',(-0.433883739117558,0.900968867902419,0.));
#14757=DIRECTION('ref_axis',(0.900968867902419,0.433883739117558,0.));
#14758=DIRECTION('center_axis',(0.,0.,1.));
#14759=DIRECTION('ref_axis',(-1.,-1.22464679914735E-16,0.));
#14760=DIRECTION('center_axis',(0.,0.,1.));
#14761=DIRECTION('ref_axis',(-1.,6.98296267768627E-15,0.));
#14762=DIRECTION('center_axis',(0.,0.,1.));
#14763=DIRECTION('ref_axis',(1.,0.,0.));
#14764=DIRECTION('center_axis',(0.,0.,1.));
#14765=DIRECTION('ref_axis',(1.,0.,0.));
#14766=DIRECTION('center_axis',(0.,0.,1.));
#14767=DIRECTION('ref_axis',(-0.900968867902419,0.433883739117559,0.));
#14768=DIRECTION('center_axis',(0.433883739117558,0.900968867902419,0.));
#14769=DIRECTION('ref_axis',(0.900968867902419,-0.433883739117558,0.));
#14770=DIRECTION('center_axis',(0.433883739117558,0.900968867902419,0.));
#14771=DIRECTION('ref_axis',(0.900968867902419,-0.433883739117558,0.));
#14772=DIRECTION('center_axis',(0.,0.,1.));
#14773=DIRECTION('ref_axis',(1.,0.,0.));
#14774=DIRECTION('center_axis',(0.,0.,1.));
#14775=DIRECTION('ref_axis',(1.,0.,0.));
#14776=DIRECTION('center_axis',(0.,0.,1.));
#14777=DIRECTION('ref_axis',(1.,0.,0.));
#14778=DIRECTION('center_axis',(0.,0.,1.));
#14779=DIRECTION('ref_axis',(-0.222520933956314,0.974927912181824,0.));
#14780=DIRECTION('center_axis',(0.974927912181824,0.222520933956314,0.));
#14781=DIRECTION('ref_axis',(0.222520933956314,-0.974927912181824,0.));
#14782=DIRECTION('center_axis',(0.974927912181824,0.222520933956314,0.));
#14783=DIRECTION('ref_axis',(0.222520933956314,-0.974927912181824,0.));
#14784=DIRECTION('center_axis',(0.,0.,1.));
#14785=DIRECTION('ref_axis',(1.,0.,0.));
#14786=DIRECTION('center_axis',(0.,0.,1.));
#14787=DIRECTION('ref_axis',(1.,0.,0.));
#14788=DIRECTION('center_axis',(0.,0.,1.));
#14789=DIRECTION('ref_axis',(1.,0.,0.));
#14790=DIRECTION('center_axis',(0.,0.,1.));
#14791=DIRECTION('ref_axis',(0.623489801858733,0.78183148246803,0.));
#14792=DIRECTION('center_axis',(0.78183148246803,-0.623489801858733,0.));
#14793=DIRECTION('ref_axis',(-0.623489801858733,-0.78183148246803,0.));
#14794=DIRECTION('center_axis',(0.78183148246803,-0.623489801858733,0.));
#14795=DIRECTION('ref_axis',(-0.623489801858733,-0.78183148246803,0.));
#14796=DIRECTION('center_axis',(0.,0.,1.));
#14797=DIRECTION('ref_axis',(1.,0.,0.));
#14798=DIRECTION('',(0.,0.,-1.));
#14799=DIRECTION('center_axis',(0.,0.,1.));
#14800=DIRECTION('ref_axis',(1.,0.,0.));
#14801=DIRECTION('center_axis',(0.,0.,1.));
#14802=DIRECTION('ref_axis',(1.,0.,0.));
#14803=DIRECTION('center_axis',(0.,0.,1.));
#14804=DIRECTION('ref_axis',(1.,0.,0.));
#14805=DIRECTION('center_axis',(0.,0.,1.));
#14806=DIRECTION('ref_axis',(1.,0.,0.));
#14807=DIRECTION('',(0.,0.,-1.));
#14808=DIRECTION('center_axis',(0.,0.,1.));
#14809=DIRECTION('ref_axis',(1.,0.,0.));
#14810=DIRECTION('center_axis',(0.,0.,1.));
#14811=DIRECTION('ref_axis',(1.,0.,0.));
#14812=DIRECTION('center_axis',(0.,0.,1.));
#14813=DIRECTION('ref_axis',(1.,0.,0.));
#14814=DIRECTION('center_axis',(0.,0.,1.));
#14815=DIRECTION('ref_axis',(1.,0.,0.));
#14816=DIRECTION('center_axis',(1.22464679914735E-16,-1.,0.));
#14817=DIRECTION('ref_axis',(-1.,-1.22464679914735E-16,0.));
#14818=DIRECTION('center_axis',(1.22464679914735E-16,-1.,0.));
#14819=DIRECTION('ref_axis',(-1.,-1.22464679914735E-16,0.));
#14820=DIRECTION('center_axis',(0.,0.,1.));
#14821=DIRECTION('ref_axis',(1.,0.,0.));
#14822=DIRECTION('center_axis',(0.,0.,-1.));
#14823=DIRECTION('ref_axis',(-1.,0.,0.));
#14824=DIRECTION('center_axis',(0.,0.,1.));
#14825=DIRECTION('ref_axis',(1.,0.,0.));
#14826=DIRECTION('center_axis',(0.,0.,1.));
#14827=DIRECTION('ref_axis',(1.,0.,0.));
#14828=DIRECTION('center_axis',(0.,0.,1.));
#14829=DIRECTION('ref_axis',(1.,0.,0.));
#14830=DIRECTION('',(0.70710678118655,8.65956056235497E-17,-0.707106781186545));
#14831=DIRECTION('center_axis',(0.,0.,1.));
#14832=DIRECTION('ref_axis',(1.,0.,0.));
#14833=DIRECTION('center_axis',(0.,0.,1.));
#14834=DIRECTION('ref_axis',(1.,0.,0.));
#14835=DIRECTION('',(0.,0.,-1.));
#14836=DIRECTION('center_axis',(0.,0.,-1.));
#14837=DIRECTION('ref_axis',(1.,0.,0.));
#14838=DIRECTION('center_axis',(0.,0.,1.));
#14839=DIRECTION('ref_axis',(1.,0.,0.));
#14840=DIRECTION('',(-0.70710678118655,-8.65956056235497E-17,-0.707106781186545));
#14841=DIRECTION('center_axis',(0.,0.,1.));
#14842=DIRECTION('ref_axis',(1.,0.,0.));
#14843=DIRECTION('center_axis',(0.,0.,1.));
#14844=DIRECTION('ref_axis',(1.,0.,0.));
#14845=DIRECTION('center_axis',(0.,0.,1.));
#14846=DIRECTION('ref_axis',(1.,0.,0.));
#14847=DIRECTION('center_axis',(0.,0.,1.));
#14848=DIRECTION('ref_axis',(1.,0.,0.));
#14849=DIRECTION('',(0.,0.,-1.));
#14850=DIRECTION('center_axis',(0.,0.,1.));
#14851=DIRECTION('ref_axis',(1.,0.,0.));
#14852=DIRECTION('center_axis',(0.,0.,-1.));
#14853=DIRECTION('ref_axis',(1.,0.,0.));
#14854=DIRECTION('',(-0.70710678118655,-8.65956056235497E-17,-0.707106781186545));
#14855=DIRECTION('center_axis',(0.,0.,1.));
#14856=DIRECTION('ref_axis',(1.,0.,0.));
#14857=DIRECTION('center_axis',(0.,0.,-1.));
#14858=DIRECTION('ref_axis',(-1.,0.,0.));
#14859=DIRECTION('center_axis',(0.,0.,1.));
#14860=DIRECTION('ref_axis',(1.,0.,0.));
#14861=DIRECTION('center_axis',(0.,0.,1.));
#14862=DIRECTION('ref_axis',(1.,0.,0.));
#14863=DIRECTION('center_axis',(0.,0.,1.));
#14864=DIRECTION('ref_axis',(1.,0.,0.));
#14865=DIRECTION('',(0.70710678118655,8.65956056235497E-17,-0.707106781186545));
#24671=CARTESIAN_POINT('',(0.,0.,0.));
#24672=CARTESIAN_POINT('Origin',(1.09,0.,3.42));
#24673=CARTESIAN_POINT('',(-1.06,-1.29812560709619E-16,3.42));
#24674=CARTESIAN_POINT('Origin',(0.,0.,3.42));
#24675=CARTESIAN_POINT('',(-0.76,-9.30731567351988E-17,3.42));
#24676=CARTESIAN_POINT('Origin',(0.,0.,3.42));
#24677=CARTESIAN_POINT('Origin',(0.76,0.,3.47));
#24678=CARTESIAN_POINT('',(-1.06,1.29812560709619E-16,3.47));
#24679=CARTESIAN_POINT('Origin',(0.,0.,3.47));
#24680=CARTESIAN_POINT('',(-0.76,-9.30731567351988E-17,3.47));
#24681=CARTESIAN_POINT('Origin',(0.,0.,3.47));
#24682=CARTESIAN_POINT('Origin',(0.,0.,3.445));
#24683=CARTESIAN_POINT('',(-0.76,-9.30731567351988E-17,3.445));
#24684=CARTESIAN_POINT('Origin',(0.,0.,3.1));
#24685=CARTESIAN_POINT('',(-1.06,-1.29812560709619E-16,3.5));
#24686=CARTESIAN_POINT('Origin',(0.,0.,3.5));
#24687=CARTESIAN_POINT('',(-1.06,-1.29812560709619E-16,3.1));
#24688=CARTESIAN_POINT('Origin',(1.09,0.,2.73));
#24689=CARTESIAN_POINT('',(-1.06,-1.29812560709619E-16,2.73));
#24690=CARTESIAN_POINT('Origin',(0.,0.,2.73));
#24691=CARTESIAN_POINT('',(-0.76,-9.30731567351988E-17,2.73));
#24692=CARTESIAN_POINT('Origin',(0.,0.,2.73));
#24693=CARTESIAN_POINT('Origin',(0.76,0.,2.78));
#24694=CARTESIAN_POINT('',(-1.06,1.29812560709619E-16,2.78));
#24695=CARTESIAN_POINT('Origin',(0.,0.,2.78));
#24696=CARTESIAN_POINT('',(-0.76,-9.30731567351988E-17,2.78));
#24697=CARTESIAN_POINT('Origin',(0.,0.,2.78));
#24698=CARTESIAN_POINT('Origin',(0.,0.,2.755));
#24699=CARTESIAN_POINT('',(-0.76,-9.30731567351988E-17,2.755));
#24700=CARTESIAN_POINT('Origin',(0.,0.,3.1));
#24701=CARTESIAN_POINT('',(0.644752300229835,-0.84136464826396,2.9246182449626));
#24702=CARTESIAN_POINT('',(0.676798995897952,-0.815808261267024,2.9246182449626));
#24703=CARTESIAN_POINT('Ctrl Pts',(0.644752300229834,-0.84136464826396,
2.9246182449626));
#24704=CARTESIAN_POINT('Ctrl Pts',(0.650287628305284,-0.837122830502141,
2.92392632269117));
#24705=CARTESIAN_POINT('Ctrl Pts',(0.655704350161558,-0.832884117923057,
2.92360435804703));
#24706=CARTESIAN_POINT('Ctrl Pts',(0.666094029778957,-0.824598624909167,
2.92360435804703));
#24707=CARTESIAN_POINT('Ctrl Pts',(0.671431802990462,-0.820260913860831,
2.92392632269117));
#24708=CARTESIAN_POINT('Ctrl Pts',(0.676798995897952,-0.815808261267023,
2.9246182449626));
#24709=CARTESIAN_POINT('',(1.05980185416667,-0.0204946311236757,2.9246182449626));
#24710=CARTESIAN_POINT('Origin',(0.,0.,2.9246182449626));
#24711=CARTESIAN_POINT('',(1.05980185416667,0.0204946311236757,2.9246182449626));
#24712=CARTESIAN_POINT('Ctrl Pts',(1.05980185416667,-0.0204946311236757,
2.9246182449626));
#24713=CARTESIAN_POINT('Ctrl Pts',(1.05993668810257,-0.013522207252662,
2.92392632269117));
#24714=CARTESIAN_POINT('Ctrl Pts',(1.06,-0.00664444950758591,2.92360435804703));
#24715=CARTESIAN_POINT('Ctrl Pts',(1.06,0.00664444950758591,2.92360435804703));
#24716=CARTESIAN_POINT('Ctrl Pts',(1.05993668810257,0.0135222072526619,
2.92392632269117));
#24717=CARTESIAN_POINT('Ctrl Pts',(1.05980185416667,0.0204946311236757,
2.9246182449626));
#24718=CARTESIAN_POINT('',(0.676798995897952,0.815808261267023,2.9246182449626));
#24719=CARTESIAN_POINT('Origin',(0.,0.,2.9246182449626));
#24720=CARTESIAN_POINT('',(0.644752300229835,0.84136464826396,2.9246182449626));
#24721=CARTESIAN_POINT('Ctrl Pts',(0.676798995897952,0.815808261267023,
2.9246182449626));
#24722=CARTESIAN_POINT('Ctrl Pts',(0.671431802990462,0.820260913860831,
2.92392632269117));
#24723=CARTESIAN_POINT('Ctrl Pts',(0.666094029778957,0.824598624909167,
2.92360435804703));
#24724=CARTESIAN_POINT('Ctrl Pts',(0.655704350161558,0.832884117923057,
2.92360435804703));
#24725=CARTESIAN_POINT('Ctrl Pts',(0.650287628305285,0.83712283050214,2.92392632269117));
#24726=CARTESIAN_POINT('Ctrl Pts',(0.644752300229835,0.84136464826396,2.9246182449626));
#24727=CARTESIAN_POINT('',(-0.215847310465459,1.03779089346786,2.9246182449626));
#24728=CARTESIAN_POINT('Origin',(0.,0.,2.9246182449626));
#24729=CARTESIAN_POINT('',(-0.255808886330142,1.0286699245504,2.9246182449626));
#24730=CARTESIAN_POINT('Ctrl Pts',(-0.215847310465459,1.03779089346786,
2.9246182449626));
#24731=CARTESIAN_POINT('Ctrl Pts',(-0.222674924486219,1.03637083656377,
2.92392632269117));
#24732=CARTESIAN_POINT('Ctrl Pts',(-0.229394330707665,1.03490211602279,
2.92360435804703));
#24733=CARTESIAN_POINT('Ctrl Pts',(-0.242350049279721,1.03194505780268,
2.92360435804703));
#24734=CARTESIAN_POINT('Ctrl Pts',(-0.249041279056074,1.03035288818974,
2.92392632269117));
#24735=CARTESIAN_POINT('Ctrl Pts',(-0.255808886330142,1.0286699245504,2.9246182449626));
#24736=CARTESIAN_POINT('',(-0.945956189565658,0.478295815811116,2.9246182449626));
#24737=CARTESIAN_POINT('Origin',(0.,0.,2.9246182449626));
#24738=CARTESIAN_POINT('',(-0.963740763933195,0.441365766607993,2.9246182449626));
#24739=CARTESIAN_POINT('Ctrl Pts',(-0.945956189565658,0.478295815811116,
2.9246182449626));
#24740=CARTESIAN_POINT('Ctrl Pts',(-0.949102892084109,0.472072381221787,
2.92392632269117));
#24741=CARTESIAN_POINT('Ctrl Pts',(-0.952144081379837,0.465903205615292,
2.92360435804703));
#24742=CARTESIAN_POINT('Ctrl Pts',(-0.957909918573291,0.453930321313932,
2.92360435804703));
#24743=CARTESIAN_POINT('Ctrl Pts',(-0.960837023771914,0.447706205701861,
2.92392632269117));
#24744=CARTESIAN_POINT('Ctrl Pts',(-0.963740763933195,0.441365766607993,
2.9246182449626));
#24745=CARTESIAN_POINT('',(-1.06,-1.29812560709619E-16,2.9246182449626));
#24746=CARTESIAN_POINT('Origin',(0.,0.,2.9246182449626));
#24747=CARTESIAN_POINT('',(-1.06,-1.29812560709619E-16,3.1));
#24748=CARTESIAN_POINT('',(-0.963740763933202,-0.441365766607979,2.9246182449626));
#24749=CARTESIAN_POINT('Origin',(0.,0.,2.9246182449626));
#24750=CARTESIAN_POINT('',(-0.945956189565651,-0.47829581581113,2.9246182449626));
#24751=CARTESIAN_POINT('Ctrl Pts',(-0.963740763933202,-0.441365766607978,
2.9246182449626));
#24752=CARTESIAN_POINT('Ctrl Pts',(-0.960837023771919,-0.447706205701851,
2.92392632269117));
#24753=CARTESIAN_POINT('Ctrl Pts',(-0.957909918573294,-0.453930321313927,
2.92360435804703));
#24754=CARTESIAN_POINT('Ctrl Pts',(-0.952144081379835,-0.465903205615296,
2.92360435804703));
#24755=CARTESIAN_POINT('Ctrl Pts',(-0.949102892084104,-0.472072381221796,
2.92392632269117));
#24756=CARTESIAN_POINT('Ctrl Pts',(-0.945956189565651,-0.47829581581113,
2.9246182449626));
#24757=CARTESIAN_POINT('',(-0.255808886330126,-1.02866992455041,2.9246182449626));
#24758=CARTESIAN_POINT('Origin',(0.,0.,2.9246182449626));
#24759=CARTESIAN_POINT('',(-0.215847310465475,-1.03779089346786,2.9246182449626));
#24760=CARTESIAN_POINT('Ctrl Pts',(-0.255808886330127,-1.02866992455041,
2.9246182449626));
#24761=CARTESIAN_POINT('Ctrl Pts',(-0.249041279056064,-1.03035288818974,
2.92392632269117));
#24762=CARTESIAN_POINT('Ctrl Pts',(-0.242350049279717,-1.03194505780268,
2.92360435804703));
#24763=CARTESIAN_POINT('Ctrl Pts',(-0.22939433070767,-1.03490211602279,
2.92360435804703));
#24764=CARTESIAN_POINT('Ctrl Pts',(-0.222674924486229,-1.03637083656377,
2.92392632269117));
#24765=CARTESIAN_POINT('Ctrl Pts',(-0.215847310465475,-1.03779089346786,
2.9246182449626));
#24766=CARTESIAN_POINT('Origin',(0.,0.,2.9246182449626));
#24767=CARTESIAN_POINT('Origin',(0.56114082167286,-0.703648334221227,3.1));
#24768=CARTESIAN_POINT('',(0.447871167131128,-0.589076750222415,3.2753817550374));
#24769=CARTESIAN_POINT('',(0.461382453375463,-0.578555297026342,3.27639564195297));
#24770=CARTESIAN_POINT('Ctrl Pts',(0.447871167131128,-0.589076750222415,
3.2753817550374));
#24771=CARTESIAN_POINT('Ctrl Pts',(0.452502352671194,-0.585555690407633,
3.27607258736419));
#24772=CARTESIAN_POINT('Ctrl Pts',(0.457039480081211,-0.582018702657134,
3.27639564195297));
#24773=CARTESIAN_POINT('Ctrl Pts',(0.461382453375463,-0.578555297026342,
3.27639564195297));
#24774=CARTESIAN_POINT('',(0.447871167131128,-0.589076750222415,2.9246182449626));
#24775=CARTESIAN_POINT('Ctrl Pts',(0.447871167131128,-0.589076750222415,
2.9246182449626));
#24776=CARTESIAN_POINT('Ctrl Pts',(0.446194419897492,-0.586923529425737,
2.92710779980363));
#24777=CARTESIAN_POINT('Ctrl Pts',(0.444580537728587,-0.584850895382108,
2.92962121790888));
#24778=CARTESIAN_POINT('Ctrl Pts',(0.436672122204369,-0.574693882270445,
2.9424934277131));
#24779=CARTESIAN_POINT('Ctrl Pts',(0.430350710191137,-0.566572846562105,
2.95482825180595));
#24780=CARTESIAN_POINT('Ctrl Pts',(0.419449625073302,-0.552565269832585,
2.98139101419695));
#24781=CARTESIAN_POINT('Ctrl Pts',(0.414869876004012,-0.546678794884774,
2.99561895616294));
#24782=CARTESIAN_POINT('Ctrl Pts',(0.407985330685283,-0.537828888858989,
3.02268687665294));
#24783=CARTESIAN_POINT('Ctrl Pts',(0.40504622519769,-0.534050030841187,
3.03802055188041));
#24784=CARTESIAN_POINT('Ctrl Pts',(0.401219893621933,-0.529130146180412,
3.06935267774138));
#24785=CARTESIAN_POINT('Ctrl Pts',(0.400332631188562,-0.52798915178784,
3.08535112900039));
#24786=CARTESIAN_POINT('Ctrl Pts',(0.400332631188562,-0.52798915178784,
3.11464887099961));
#24787=CARTESIAN_POINT('Ctrl Pts',(0.401219893621933,-0.529130146180413,
3.13064732225863));
#24788=CARTESIAN_POINT('Ctrl Pts',(0.40504622519769,-0.534050030841188,
3.16197944811959));
#24789=CARTESIAN_POINT('Ctrl Pts',(0.407985330685283,-0.537828888858989,
3.17731312334706));
#24790=CARTESIAN_POINT('Ctrl Pts',(0.414869876004012,-0.546678794884774,
3.20438104383706));
#24791=CARTESIAN_POINT('Ctrl Pts',(0.419449625073302,-0.552565269832586,
3.21860898580305));
#24792=CARTESIAN_POINT('Ctrl Pts',(0.430350710191136,-0.566572846562106,
3.24517174819405));
#24793=CARTESIAN_POINT('Ctrl Pts',(0.436672122204372,-0.574693882270443,
3.2575065722869));
#24794=CARTESIAN_POINT('Ctrl Pts',(0.44458053772859,-0.584850895382106,
3.27037878209112));
#24795=CARTESIAN_POINT('Ctrl Pts',(0.446194419897492,-0.586923529425737,
3.27289220019637));
#24796=CARTESIAN_POINT('Ctrl Pts',(0.447871167131128,-0.589076750222415,
3.2753817550374));
#24797=CARTESIAN_POINT('',(0.461382453375463,-0.578555297026342,2.92360435804703));
#24798=CARTESIAN_POINT('Ctrl Pts',(0.461382453375463,-0.578555297026342,
2.92360435804703));
#24799=CARTESIAN_POINT('Ctrl Pts',(0.457039480081211,-0.582018702657134,
2.92360435804703));
#24800=CARTESIAN_POINT('Ctrl Pts',(0.452502352671194,-0.585555690407633,
2.92392741263581));
#24801=CARTESIAN_POINT('Ctrl Pts',(0.447871167131128,-0.589076750222415,
2.9246182449626));
#24802=CARTESIAN_POINT('',(0.56114082167286,-0.703648334221227,2.86185));
#24803=CARTESIAN_POINT('Origin',(0.56114082167286,-0.703648334221227,3.1));
#24804=CARTESIAN_POINT('',(0.474646655807069,-0.56772401052903,2.9246182449626));
#24805=CARTESIAN_POINT('Ctrl Pts',(0.474646655807069,-0.56772401052903,
2.9246182449626));
#24806=CARTESIAN_POINT('Ctrl Pts',(0.470183340581476,-0.571455573060032,
2.92392741263581));
#24807=CARTESIAN_POINT('Ctrl Pts',(0.465725426669714,-0.57509189139555,
2.92360435804703));
#24808=CARTESIAN_POINT('Ctrl Pts',(0.461382453375463,-0.578555297026342,
2.92360435804703));
#24809=CARTESIAN_POINT('',(0.474646655807069,-0.56772401052903,3.2753817550374));
#24810=CARTESIAN_POINT('Ctrl Pts',(0.474646655807069,-0.56772401052903,
3.2753817550374));
#24811=CARTESIAN_POINT('Ctrl Pts',(0.472920532111735,-0.565610166146593,
3.27289220019637));
#24812=CARTESIAN_POINT('Ctrl Pts',(0.47125898589838,-0.56357554291002,3.27037878209112));
#24813=CARTESIAN_POINT('Ctrl Pts',(0.463116418319987,-0.553605259830513,
3.2575065722869));
#24814=CARTESIAN_POINT('Ctrl Pts',(0.456605640437212,-0.545635238363897,
3.24517174819405));
#24815=CARTESIAN_POINT('Ctrl Pts',(0.445374982543132,-0.531890487153133,
3.21860898580305));
#24816=CARTESIAN_POINT('Ctrl Pts',(0.440655183852335,-0.526115698051596,
3.20438104383706));
#24817=CARTESIAN_POINT('Ctrl Pts',(0.433559118901799,-0.517434473303403,
3.17731312334706));
#24818=CARTESIAN_POINT('Ctrl Pts',(0.430529017242169,-0.513728182311292,
3.16197944811959));
#24819=CARTESIAN_POINT('Ctrl Pts',(0.426583923237528,-0.50890300752715,
3.13064732225863));
#24820=CARTESIAN_POINT('Ctrl Pts',(0.425668970421903,-0.507784095477554,
3.11464887099961));
#24821=CARTESIAN_POINT('Ctrl Pts',(0.425668970421903,-0.507784095477554,
3.08535112900039));
#24822=CARTESIAN_POINT('Ctrl Pts',(0.426583923237527,-0.508903007527151,
3.06935267774138));
#24823=CARTESIAN_POINT('Ctrl Pts',(0.430529017242168,-0.513728182311292,
3.03802055188041));
#24824=CARTESIAN_POINT('Ctrl Pts',(0.433559118901799,-0.517434473303403,
3.02268687665294));
#24825=CARTESIAN_POINT('Ctrl Pts',(0.440655183852335,-0.526115698051596,
2.99561895616294));
#24826=CARTESIAN_POINT('Ctrl Pts',(0.445374982543132,-0.531890487153132,
2.98139101419695));
#24827=CARTESIAN_POINT('Ctrl Pts',(0.456605640437212,-0.545635238363897,
2.95482825180595));
#24828=CARTESIAN_POINT('Ctrl Pts',(0.463116418319989,-0.553605259830511,
2.9424934277131));
#24829=CARTESIAN_POINT('Ctrl Pts',(0.471258985898383,-0.563575542910017,
2.92962121790888));
#24830=CARTESIAN_POINT('Ctrl Pts',(0.472920532111735,-0.565610166146593,
2.92710779980363));
#24831=CARTESIAN_POINT('Ctrl Pts',(0.474646655807069,-0.56772401052903,
2.9246182449626));
#24832=CARTESIAN_POINT('Ctrl Pts',(0.461382453375463,-0.578555297026342,
3.27639564195297));
#24833=CARTESIAN_POINT('Ctrl Pts',(0.465725426669714,-0.57509189139555,
3.27639564195297));
#24834=CARTESIAN_POINT('Ctrl Pts',(0.470183340581476,-0.571455573060032,
3.27607258736419));
#24835=CARTESIAN_POINT('Ctrl Pts',(0.474646655807069,-0.56772401052903,
3.2753817550374));
#24836=CARTESIAN_POINT('',(0.56114082167286,-0.703648334221227,3.33815));
#24837=CARTESIAN_POINT('Origin',(0.56114082167286,-0.703648334221227,3.1));
#24838=CARTESIAN_POINT('',(0.644752300229835,-0.84136464826396,3.2753817550374));
#24839=CARTESIAN_POINT('Ctrl Pts',(0.644752300229835,-0.84136464826396,
3.2753817550374));
#24840=CARTESIAN_POINT('Ctrl Pts',(0.646433000359351,-0.843514492555987,
3.27289236009202));
#24841=CARTESIAN_POINT('Ctrl Pts',(0.648050798688572,-0.845583794128261,
3.27037910645452));
#24842=CARTESIAN_POINT('Ctrl Pts',(0.655979290360836,-0.85572466858529,
3.25750707214144));
#24843=CARTESIAN_POINT('Ctrl Pts',(0.662318522702308,-0.863831545066573,
3.24517226455888));
#24844=CARTESIAN_POINT('Ctrl Pts',(0.673252578886601,-0.877812903896684,
3.21860957458692));
#24845=CARTESIAN_POINT('Ctrl Pts',(0.677847358284485,-0.883687417317991,
3.2043816902577));
#24846=CARTESIAN_POINT('Ctrl Pts',(0.684755270452365,-0.892518849463665,
3.17731372034463));
#24847=CARTESIAN_POINT('Ctrl Pts',(0.687704871914685,-0.8962894383426,3.16197991083841));
#24848=CARTESIAN_POINT('Ctrl Pts',(0.691545075614567,-0.901198384221383,
3.13064753590579));
#24849=CARTESIAN_POINT('Ctrl Pts',(0.692435660859823,-0.902336752864262,
3.11464897022091));
#24850=CARTESIAN_POINT('Ctrl Pts',(0.692435660859823,-0.902336752864262,
3.1));
#24851=CARTESIAN_POINT('Ctrl Pts',(0.692435660859823,-0.902336752864262,
3.08535102977909));
#24852=CARTESIAN_POINT('Ctrl Pts',(0.691545075614567,-0.901198384221384,
3.06935246409421));
#24853=CARTESIAN_POINT('Ctrl Pts',(0.687704871914684,-0.896289438342601,
3.03802008916159));
#24854=CARTESIAN_POINT('Ctrl Pts',(0.684755270452365,-0.892518849463665,
3.02268627965537));
#24855=CARTESIAN_POINT('Ctrl Pts',(0.677847358284485,-0.883687417317991,
2.9956183097423));
#24856=CARTESIAN_POINT('Ctrl Pts',(0.6732525788866,-0.877812903896685,2.98139042541308));
#24857=CARTESIAN_POINT('Ctrl Pts',(0.662318522702306,-0.863831545066573,
2.95482773544112));
#24858=CARTESIAN_POINT('Ctrl Pts',(0.655979290360836,-0.85572466858529,
2.94249292785856));
#24859=CARTESIAN_POINT('Ctrl Pts',(0.648050798688553,-0.845583794128238,
2.92962089354545));
#24860=CARTESIAN_POINT('Ctrl Pts',(0.646433000359338,-0.84351449255597,
2.92710763990797));
#24861=CARTESIAN_POINT('Ctrl Pts',(0.644752300229835,-0.84136464826396,
2.9246182449626));
#24862=CARTESIAN_POINT('',(0.676798995897952,-0.815808261267024,3.2753817550374));
#24863=CARTESIAN_POINT('Ctrl Pts',(0.676798995897952,-0.815808261267023,
3.2753817550374));
#24864=CARTESIAN_POINT('Ctrl Pts',(0.671431802990462,-0.820260913860831,
3.27607367730883));
#24865=CARTESIAN_POINT('Ctrl Pts',(0.666094029778957,-0.824598624909167,
3.27639564195297));
#24866=CARTESIAN_POINT('Ctrl Pts',(0.655704350161557,-0.832884117923057,
3.27639564195297));
#24867=CARTESIAN_POINT('Ctrl Pts',(0.650287628305284,-0.837122830502141,
3.27607367730883));
#24868=CARTESIAN_POINT('Ctrl Pts',(0.644752300229834,-0.84136464826396,
3.2753817550374));
#24869=CARTESIAN_POINT('Ctrl Pts',(0.676798995897952,-0.815808261267024,
2.9246182449626));
#24870=CARTESIAN_POINT('Ctrl Pts',(0.678520948142573,-0.817925208095019,
2.92710763990798));
#24871=CARTESIAN_POINT('Ctrl Pts',(0.680178374008934,-0.819962907760957,
2.92962089354548));
#24872=CARTESIAN_POINT('Ctrl Pts',(0.688300740199246,-0.829949172449061,
2.94249292785856));
#24873=CARTESIAN_POINT('Ctrl Pts',(0.694793748460268,-0.837933416726651,
2.95482773544112));
#24874=CARTESIAN_POINT('Ctrl Pts',(0.705991509039913,-0.851704478318938,
2.98139042541308));
#24875=CARTESIAN_POINT('Ctrl Pts',(0.710696301541893,-0.8574912592173,2.9956183097423));
#24876=CARTESIAN_POINT('Ctrl Pts',(0.717769156177965,-0.866191154133894,
3.02268627965537));
#24877=CARTESIAN_POINT('Ctrl Pts',(0.720788860449205,-0.86990583788823,
3.03802008916159));
#24878=CARTESIAN_POINT('Ctrl Pts',(0.72472020309194,-0.874742102885397,
3.06935246409421));
#24879=CARTESIAN_POINT('Ctrl Pts',(0.725631856595695,-0.875863670152773,
3.08535102977909));
#24880=CARTESIAN_POINT('Ctrl Pts',(0.725631856595695,-0.875863670152773,
3.1));
#24881=CARTESIAN_POINT('Ctrl Pts',(0.725631856595695,-0.875863670152773,
3.11464897022091));
#24882=CARTESIAN_POINT('Ctrl Pts',(0.724720203091942,-0.874742102885395,
3.13064753590579));
#24883=CARTESIAN_POINT('Ctrl Pts',(0.720788860449207,-0.869905837888228,
3.16197991083841));
#24884=CARTESIAN_POINT('Ctrl Pts',(0.717769156177965,-0.866191154133894,
3.17731372034463));
#24885=CARTESIAN_POINT('Ctrl Pts',(0.710696301541893,-0.8574912592173,3.2043816902577));
#24886=CARTESIAN_POINT('Ctrl Pts',(0.705991509039915,-0.851704478318937,
3.21860957458692));
#24887=CARTESIAN_POINT('Ctrl Pts',(0.694793748460269,-0.83793341672665,
3.24517226455888));
#24888=CARTESIAN_POINT('Ctrl Pts',(0.688300740199246,-0.829949172449061,
3.25750707214144));
#24889=CARTESIAN_POINT('Ctrl Pts',(0.680178374008915,-0.819962907760934,
3.27037910645455));
#24890=CARTESIAN_POINT('Ctrl Pts',(0.678520948142559,-0.817925208095002,
3.27289236009204));
#24891=CARTESIAN_POINT('Ctrl Pts',(0.676798995897952,-0.815808261267024,
3.2753817550374));
#24892=CARTESIAN_POINT('Origin',(0.,0.,3.1));
#24893=CARTESIAN_POINT('',(-1.06,-1.29812560709619E-16,3.2753817550374));
#24894=CARTESIAN_POINT('',(-1.06,-1.29812560709619E-16,3.1));
#24895=CARTESIAN_POINT('',(-0.963740763933206,0.441365766607969,3.2753817550374));
#24896=CARTESIAN_POINT('Origin',(0.,0.,3.2753817550374));
#24897=CARTESIAN_POINT('',(-0.945956189565646,0.47829581581114,3.2753817550374));
#24898=CARTESIAN_POINT('Ctrl Pts',(-0.963740763933206,0.441365766607969,
3.2753817550374));
#24899=CARTESIAN_POINT('Ctrl Pts',(-0.960837023771922,0.447706205701845,
3.27607367730883));
#24900=CARTESIAN_POINT('Ctrl Pts',(-0.957909918573295,0.453930321313924,
3.27639564195297));
#24901=CARTESIAN_POINT('Ctrl Pts',(-0.952144081379834,0.465903205615299,
3.27639564195297));
#24902=CARTESIAN_POINT('Ctrl Pts',(-0.949102892084101,0.472072381221803,
3.27607367730883));
#24903=CARTESIAN_POINT('Ctrl Pts',(-0.945956189565646,0.47829581581114,
3.2753817550374));
#24904=CARTESIAN_POINT('',(-0.255808886330142,1.0286699245504,3.2753817550374));
#24905=CARTESIAN_POINT('Origin',(0.,0.,3.2753817550374));
#24906=CARTESIAN_POINT('',(-0.215847310465459,1.03779089346786,3.2753817550374));
#24907=CARTESIAN_POINT('Ctrl Pts',(-0.255808886330142,1.0286699245504,3.2753817550374));
#24908=CARTESIAN_POINT('Ctrl Pts',(-0.249041279056074,1.03035288818974,
3.27607367730883));
#24909=CARTESIAN_POINT('Ctrl Pts',(-0.242350049279721,1.03194505780268,
3.27639564195297));
#24910=CARTESIAN_POINT('Ctrl Pts',(-0.229394330707665,1.03490211602279,
3.27639564195297));
#24911=CARTESIAN_POINT('Ctrl Pts',(-0.222674924486219,1.03637083656377,
3.27607367730883));
#24912=CARTESIAN_POINT('Ctrl Pts',(-0.215847310465459,1.03779089346786,
3.2753817550374));
#24913=CARTESIAN_POINT('',(0.644752300229835,0.84136464826396,3.2753817550374));
#24914=CARTESIAN_POINT('Origin',(0.,0.,3.2753817550374));
#24915=CARTESIAN_POINT('',(0.676798995897952,0.815808261267023,3.2753817550374));
#24916=CARTESIAN_POINT('Ctrl Pts',(0.644752300229835,0.84136464826396,3.2753817550374));
#24917=CARTESIAN_POINT('Ctrl Pts',(0.650287628305285,0.83712283050214,3.27607367730883));
#24918=CARTESIAN_POINT('Ctrl Pts',(0.655704350161558,0.832884117923057,
3.27639564195297));
#24919=CARTESIAN_POINT('Ctrl Pts',(0.666094029778957,0.824598624909166,
3.27639564195297));
#24920=CARTESIAN_POINT('Ctrl Pts',(0.671431802990462,0.82026091386083,3.27607367730883));
#24921=CARTESIAN_POINT('Ctrl Pts',(0.676798995897952,0.815808261267023,
3.2753817550374));
#24922=CARTESIAN_POINT('',(1.05980185416667,0.0204946311236757,3.2753817550374));
#24923=CARTESIAN_POINT('Origin',(0.,0.,3.2753817550374));
#24924=CARTESIAN_POINT('',(1.05980185416667,-0.0204946311236757,3.2753817550374));
#24925=CARTESIAN_POINT('Ctrl Pts',(1.05980185416667,0.0204946311236757,
3.2753817550374));
#24926=CARTESIAN_POINT('Ctrl Pts',(1.05993668810257,0.0135222072526619,
3.27607367730883));
#24927=CARTESIAN_POINT('Ctrl Pts',(1.06,0.00664444950758593,3.27639564195297));
#24928=CARTESIAN_POINT('Ctrl Pts',(1.06,-0.0066444495075859,3.27639564195297));
#24929=CARTESIAN_POINT('Ctrl Pts',(1.05993668810257,-0.013522207252662,
3.27607367730883));
#24930=CARTESIAN_POINT('Ctrl Pts',(1.05980185416667,-0.0204946311236757,
3.2753817550374));
#24931=CARTESIAN_POINT('Origin',(0.,0.,3.2753817550374));
#24932=CARTESIAN_POINT('',(-0.215847310465448,-1.03779089346787,3.2753817550374));
#24933=CARTESIAN_POINT('Origin',(0.,0.,3.2753817550374));
#24934=CARTESIAN_POINT('',(-0.255808886330153,-1.0286699245504,3.2753817550374));
#24935=CARTESIAN_POINT('Ctrl Pts',(-0.215847310465448,-1.03779089346787,
3.2753817550374));
#24936=CARTESIAN_POINT('Ctrl Pts',(-0.222674924486212,-1.03637083656377,
3.27607367730883));
#24937=CARTESIAN_POINT('Ctrl Pts',(-0.229394330707662,-1.03490211602279,
3.27639564195297));
#24938=CARTESIAN_POINT('Ctrl Pts',(-0.242350049279725,-1.03194505780268,
3.27639564195297));
#24939=CARTESIAN_POINT('Ctrl Pts',(-0.249041279056081,-1.03035288818974,
3.27607367730883));
#24940=CARTESIAN_POINT('Ctrl Pts',(-0.255808886330153,-1.0286699245504,
3.2753817550374));
#24941=CARTESIAN_POINT('',(-0.945956189565651,-0.47829581581113,3.2753817550374));
#24942=CARTESIAN_POINT('Origin',(0.,0.,3.2753817550374));
#24943=CARTESIAN_POINT('',(-0.963740763933202,-0.441365766607979,3.2753817550374));
#24944=CARTESIAN_POINT('Ctrl Pts',(-0.945956189565651,-0.47829581581113,
3.2753817550374));
#24945=CARTESIAN_POINT('Ctrl Pts',(-0.949102892084104,-0.472072381221796,
3.27607367730883));
#24946=CARTESIAN_POINT('Ctrl Pts',(-0.952144081379835,-0.465903205615296,
3.27639564195297));
#24947=CARTESIAN_POINT('Ctrl Pts',(-0.957909918573294,-0.453930321313927,
3.27639564195297));
#24948=CARTESIAN_POINT('Ctrl Pts',(-0.960837023771919,-0.447706205701851,
3.27607367730883));
#24949=CARTESIAN_POINT('Ctrl Pts',(-0.963740763933202,-0.441365766607978,
3.2753817550374));
#24950=CARTESIAN_POINT('Origin',(0.,0.,3.2753817550374));
#24951=CARTESIAN_POINT('Origin',(0.,0.,3.1));
#24952=CARTESIAN_POINT('Ctrl Pts',(-0.215847310465468,-1.03779089346786,
2.9246182449626));
#24953=CARTESIAN_POINT('Ctrl Pts',(-0.216428786478497,-1.04045706470235,
2.92710763990799));
#24954=CARTESIAN_POINT('Ctrl Pts',(-0.21698853610412,-1.04302337738549,
2.92962089354548));
#24955=CARTESIAN_POINT('Ctrl Pts',(-0.219731899742916,-1.0556000331769,
2.94249292785856));
#24956=CARTESIAN_POINT('Ctrl Pts',(-0.221925908848724,-1.06565456633392,
2.95482773544113));
#24957=CARTESIAN_POINT('Ctrl Pts',(-0.225710868823514,-1.08299544455179,
2.98139042541308));
#24958=CARTESIAN_POINT('Ctrl Pts',(-0.227301766167146,-1.09028179832404,
2.9956183097423));
#24959=CARTESIAN_POINT('Ctrl Pts',(-0.229693765171481,-1.10123587450718,
3.02268627965537));
#24960=CARTESIAN_POINT('Ctrl Pts',(-0.230715267060294,-1.10591284181213,
3.03802008916159));
#24961=CARTESIAN_POINT('Ctrl Pts',(-0.232045259247278,-1.11200185116341,
3.06935246409421));
#24962=CARTESIAN_POINT('Ctrl Pts',(-0.232353729184198,-1.11341389632706,
3.08535102977909));
#24963=CARTESIAN_POINT('Ctrl Pts',(-0.232353729184197,-1.11341389632706,
3.1));
#24964=CARTESIAN_POINT('Ctrl Pts',(-0.232353729184196,-1.11341389632706,
3.11464897022091));
#24965=CARTESIAN_POINT('Ctrl Pts',(-0.232045259247272,-1.11200185116341,
3.13064753590579));
#24966=CARTESIAN_POINT('Ctrl Pts',(-0.230715267060285,-1.10591284181213,
3.16197991083841));
#24967=CARTESIAN_POINT('Ctrl Pts',(-0.229693765171472,-1.10123587450718,
3.17731372034463));
#24968=CARTESIAN_POINT('Ctrl Pts',(-0.227301766167134,-1.09028179832404,
3.2043816902577));
#24969=CARTESIAN_POINT('Ctrl Pts',(-0.225710868823502,-1.08299544455179,
3.21860957458692));
#24970=CARTESIAN_POINT('Ctrl Pts',(-0.221925908848709,-1.06565456633392,
3.24517226455888));
#24971=CARTESIAN_POINT('Ctrl Pts',(-0.219731899742906,-1.05560003317691,
3.25750707214144));
#24972=CARTESIAN_POINT('Ctrl Pts',(-0.216988536104103,-1.04302337738546,
3.27037910645455));
#24973=CARTESIAN_POINT('Ctrl Pts',(-0.216428786478473,-1.04045706470233,
3.27289236009203));
#24974=CARTESIAN_POINT('Ctrl Pts',(-0.215847310465448,-1.03779089346787,
3.2753817550374));
#24975=CARTESIAN_POINT('Origin',(0.,0.,3.1));
#24976=CARTESIAN_POINT('',(-0.147927155402556,-0.725063829393322,2.9246182449626));
#24977=CARTESIAN_POINT('Origin',(0.,0.,2.9246182449626));
#24978=CARTESIAN_POINT('',(-0.164665491127673,-0.72144665501455,2.92360435804703));
#24979=CARTESIAN_POINT('Ctrl Pts',(-0.147927155402556,-0.725063829393322,
2.9246182449626));
#24980=CARTESIAN_POINT('Ctrl Pts',(-0.153627439993726,-0.723900860216853,
2.92392741263581));
#24981=CARTESIAN_POINT('Ctrl Pts',(-0.159249892010255,-0.722682730173013,
2.92360435804703));
#24982=CARTESIAN_POINT('Ctrl Pts',(-0.164665491127673,-0.72144665501455,
2.92360435804703));
#24983=CARTESIAN_POINT('',(-0.181315643661004,-0.717443124828579,2.9246182449626));
#24984=CARTESIAN_POINT('Ctrl Pts',(-0.164665491127673,-0.72144665501455,
2.92360435804703));
#24985=CARTESIAN_POINT('Ctrl Pts',(-0.170081090245091,-0.720210579856086,
2.92360435804703));
#24986=CARTESIAN_POINT('Ctrl Pts',(-0.175675271291411,-0.718868586598702,
2.92392741263581));
#24987=CARTESIAN_POINT('Ctrl Pts',(-0.181315643661004,-0.717443124828579,
2.9246182449626));
#24988=CARTESIAN_POINT('',(-0.659108801429989,-0.336415796117726,2.9246182449626));
#24989=CARTESIAN_POINT('Origin',(0.,0.,2.9246182449626));
#24990=CARTESIAN_POINT('',(-0.66671696224779,-0.321073966946993,2.92360435804703));
#24991=CARTESIAN_POINT('Ctrl Pts',(-0.659108801429989,-0.336415796117726,
2.9246182449626));
#24992=CARTESIAN_POINT('Ctrl Pts',(-0.661753624824974,-0.331234034743915,
2.92392741263581));
#24993=CARTESIAN_POINT('Ctrl Pts',(-0.664306793900707,-0.326078733089052,
2.92360435804703));
#24994=CARTESIAN_POINT('Ctrl Pts',(-0.66671696224779,-0.321073966946993,
2.92360435804703));
#24995=CARTESIAN_POINT('',(-0.673968076611316,-0.305560193266145,2.9246182449626));
#24996=CARTESIAN_POINT('Ctrl Pts',(-0.66671696224779,-0.321073966946993,
2.92360435804703));
#24997=CARTESIAN_POINT('Ctrl Pts',(-0.669127130594873,-0.316069200804934,
2.92360435804703));
#24998=CARTESIAN_POINT('Ctrl Pts',(-0.671565832849124,-0.310858774834149,
2.92392741263581));
#24999=CARTESIAN_POINT('Ctrl Pts',(-0.673968076611316,-0.305560193266145,
2.9246182449626));
#25000=CARTESIAN_POINT('',(-0.74,-9.06238631369041E-17,2.9246182449626));
#25001=CARTESIAN_POINT('Origin',(0.,0.,2.9246182449626));
#25002=CARTESIAN_POINT('',(-0.74,-9.06238631369041E-17,2.7));
#25003=CARTESIAN_POINT('',(-0.74,-9.06238631369041E-17,3.1));
#25004=CARTESIAN_POINT('Origin',(0.,0.,2.7));
#25005=CARTESIAN_POINT('',(-0.673968076611311,0.305560193266154,2.9246182449626));
#25006=CARTESIAN_POINT('Origin',(0.,0.,2.9246182449626));
#25007=CARTESIAN_POINT('',(-0.66671696224779,0.321073966946993,2.92360435804703));
#25008=CARTESIAN_POINT('Ctrl Pts',(-0.673968076611311,0.305560193266154,
2.9246182449626));
#25009=CARTESIAN_POINT('Ctrl Pts',(-0.671565832849121,0.310858774834155,
2.92392741263581));
#25010=CARTESIAN_POINT('Ctrl Pts',(-0.669127130594872,0.316069200804937,
2.92360435804703));
#25011=CARTESIAN_POINT('Ctrl Pts',(-0.66671696224779,0.321073966946993,
2.92360435804703));
#25012=CARTESIAN_POINT('',(-0.659108801429993,0.336415796117718,2.9246182449626));
#25013=CARTESIAN_POINT('Ctrl Pts',(-0.66671696224779,0.321073966946993,
2.92360435804703));
#25014=CARTESIAN_POINT('Ctrl Pts',(-0.664306793900708,0.32607873308905,
2.92360435804703));
#25015=CARTESIAN_POINT('Ctrl Pts',(-0.661753624824977,0.331234034743909,
2.92392741263581));
#25016=CARTESIAN_POINT('Ctrl Pts',(-0.659108801429993,0.336415796117718,
2.9246182449626));
#25017=CARTESIAN_POINT('',(-0.181315643661013,0.717443124828577,2.9246182449626));
#25018=CARTESIAN_POINT('Origin',(0.,0.,2.9246182449626));
#25019=CARTESIAN_POINT('',(-0.164665491127673,0.72144665501455,2.92360435804703));
#25020=CARTESIAN_POINT('Ctrl Pts',(-0.181315643661013,0.717443124828577,
2.9246182449626));
#25021=CARTESIAN_POINT('Ctrl Pts',(-0.175675271291417,0.7188685865987,2.92392741263581));
#25022=CARTESIAN_POINT('Ctrl Pts',(-0.170081090245093,0.720210579856085,
2.92360435804703));
#25023=CARTESIAN_POINT('Ctrl Pts',(-0.164665491127673,0.72144665501455,
2.92360435804703));
#25024=CARTESIAN_POINT('',(-0.147927155402546,0.725063829393324,2.9246182449626));
#25025=CARTESIAN_POINT('Ctrl Pts',(-0.164665491127673,0.72144665501455,
2.92360435804703));
#25026=CARTESIAN_POINT('Ctrl Pts',(-0.159249892010252,0.722682730173014,
2.92360435804703));
#25027=CARTESIAN_POINT('Ctrl Pts',(-0.15362743999372,0.723900860216854,
2.92392741263581));
#25028=CARTESIAN_POINT('Ctrl Pts',(-0.147927155402546,0.725063829393324,
2.9246182449626));
#25029=CARTESIAN_POINT('',(0.447871167131128,0.589076750222415,2.9246182449626));
#25030=CARTESIAN_POINT('Origin',(0.,0.,2.9246182449626));
#25031=CARTESIAN_POINT('',(0.461382453375463,0.578555297026342,2.92360435804703));
#25032=CARTESIAN_POINT('Ctrl Pts',(0.447871167131128,0.589076750222415,
2.9246182449626));
#25033=CARTESIAN_POINT('Ctrl Pts',(0.452502352671194,0.585555690407633,
2.92392741263581));
#25034=CARTESIAN_POINT('Ctrl Pts',(0.457039480081212,0.582018702657134,
2.92360435804703));
#25035=CARTESIAN_POINT('Ctrl Pts',(0.461382453375463,0.578555297026342,
2.92360435804703));
#25036=CARTESIAN_POINT('',(0.474646655807069,0.56772401052903,2.9246182449626));
#25037=CARTESIAN_POINT('Ctrl Pts',(0.461382453375463,0.578555297026342,
2.92360435804703));
#25038=CARTESIAN_POINT('Ctrl Pts',(0.465725426669714,0.57509189139555,2.92360435804703));
#25039=CARTESIAN_POINT('Ctrl Pts',(0.470183340581476,0.571455573060032,
2.92392741263581));
#25040=CARTESIAN_POINT('Ctrl Pts',(0.474646655807069,0.56772401052903,2.9246182449626));
#25041=CARTESIAN_POINT('',(0.739801854166667,0.0171235677229433,2.9246182449626));
#25042=CARTESIAN_POINT('Origin',(0.,0.,2.9246182449626));
#25043=CARTESIAN_POINT('',(0.74,-1.06645361311672E-17,2.92360435804703));
#25044=CARTESIAN_POINT('Ctrl Pts',(0.739801854166667,0.0171235677229433,
2.9246182449626));
#25045=CARTESIAN_POINT('Ctrl Pts',(0.739936475706564,0.0113074161803183,
2.92392741263581));
#25046=CARTESIAN_POINT('Ctrl Pts',(0.74,0.00555487133946257,2.92360435804703));
#25047=CARTESIAN_POINT('Ctrl Pts',(0.74,-1.73472347597681E-18,2.92360435804703));
#25048=CARTESIAN_POINT('',(0.739801854166667,-0.0171235677229433,2.9246182449626));
#25049=CARTESIAN_POINT('Ctrl Pts',(0.74,-1.73472347597681E-18,2.92360435804703));
#25050=CARTESIAN_POINT('Ctrl Pts',(0.74,-0.00555487133946261,2.92360435804703));
#25051=CARTESIAN_POINT('Ctrl Pts',(0.739936475706564,-0.0113074161803182,
2.92392741263581));
#25052=CARTESIAN_POINT('Ctrl Pts',(0.739801854166667,-0.0171235677229433,
2.9246182449626));
#25053=CARTESIAN_POINT('Origin',(0.,0.,2.9246182449626));
#25054=CARTESIAN_POINT('Origin',(0.,0.,3.1));
#25055=CARTESIAN_POINT('',(-0.147927155402543,-0.725063829393324,3.2753817550374));
#25056=CARTESIAN_POINT('Origin',(0.,0.,3.2753817550374));
#25057=CARTESIAN_POINT('Ctrl Pts',(-0.147927155402542,-0.725063829393325,
3.2753817550374));
#25058=CARTESIAN_POINT('Ctrl Pts',(-0.147350705836102,-0.722396331130513,
3.27289220019637));
#25059=CARTESIAN_POINT('Ctrl Pts',(-0.14679593045413,-0.719828715152708,
3.27037878209112));
#25060=CARTESIAN_POINT('Ctrl Pts',(-0.144077657099528,-0.70724622965008,
3.2575065722869));
#25061=CARTESIAN_POINT('Ctrl Pts',(-0.141905847013061,-0.697186671420939,
3.24517174819405));
#25062=CARTESIAN_POINT('Ctrl Pts',(-0.138161968462919,-0.679836477301522,
3.21860898580305));
#25063=CARTESIAN_POINT('Ctrl Pts',(-0.136589802889265,-0.672545867981452,
3.20438104383706));
#25064=CARTESIAN_POINT('Ctrl Pts',(-0.134226872204735,-0.661585285903343,
3.17731312334706));
#25065=CARTESIAN_POINT('Ctrl Pts',(-0.133218414707289,-0.656905422394463,
3.16197944811959));
#25066=CARTESIAN_POINT('Ctrl Pts',(-0.131905667031905,-0.650812576430241,
3.13064732225862));
#25067=CARTESIAN_POINT('Ctrl Pts',(-0.131601330115138,-0.649399607261913,
3.11464887099961));
#25068=CARTESIAN_POINT('Ctrl Pts',(-0.131601330115139,-0.649399607261913,
3.08535112900039));
#25069=CARTESIAN_POINT('Ctrl Pts',(-0.131905667031907,-0.650812576430241,
3.06935267774137));
#25070=CARTESIAN_POINT('Ctrl Pts',(-0.133218414707293,-0.656905422394462,
3.03802055188041));
#25071=CARTESIAN_POINT('Ctrl Pts',(-0.134226872204739,-0.661585285903342,
3.02268687665294));
#25072=CARTESIAN_POINT('Ctrl Pts',(-0.136589802889271,-0.672545867981451,
2.99561895616294));
#25073=CARTESIAN_POINT('Ctrl Pts',(-0.138161968462926,-0.679836477301521,
2.98139101419695));
#25074=CARTESIAN_POINT('Ctrl Pts',(-0.14190584701307,-0.697186671420938,
2.95482825180595));
#25075=CARTESIAN_POINT('Ctrl Pts',(-0.144077657099543,-0.707246229650077,
2.9424934277131));
#25076=CARTESIAN_POINT('Ctrl Pts',(-0.146795930454146,-0.719828715152705,
2.92962121790888));
#25077=CARTESIAN_POINT('Ctrl Pts',(-0.147350705836117,-0.72239633113051,
2.92710779980363));
#25078=CARTESIAN_POINT('Ctrl Pts',(-0.147927155402556,-0.725063829393322,
2.9246182449626));
#25079=CARTESIAN_POINT('Origin',(-0.200268840560683,-0.877435120963641,
3.1));
#25080=CARTESIAN_POINT('',(-0.181315643661016,-0.717443124828576,3.2753817550374));
#25081=CARTESIAN_POINT('',(-0.164665491127673,-0.72144665501455,3.27639564195297));
#25082=CARTESIAN_POINT('Ctrl Pts',(-0.181315643661016,-0.717443124828576,
3.2753817550374));
#25083=CARTESIAN_POINT('Ctrl Pts',(-0.175675271291419,-0.7188685865987,
3.27607258736419));
#25084=CARTESIAN_POINT('Ctrl Pts',(-0.170081090245095,-0.720210579856085,
3.27639564195297));
#25085=CARTESIAN_POINT('Ctrl Pts',(-0.164665491127673,-0.72144665501455,
3.27639564195297));
#25086=CARTESIAN_POINT('Ctrl Pts',(-0.181315643661004,-0.717443124828579,
2.9246182449626));
#25087=CARTESIAN_POINT('Ctrl Pts',(-0.180677622653924,-0.714789679845302,
2.92710779980363));
#25088=CARTESIAN_POINT('Ctrl Pts',(-0.180063411180689,-0.712235629767472,
2.92962121790888));
#25089=CARTESIAN_POINT('Ctrl Pts',(-0.177053154990362,-0.699719787441732,
2.9424934277131));
#25090=CARTESIAN_POINT('Ctrl Pts',(-0.174645209526939,-0.689714125571454,
2.95482825180595));
#25091=CARTESIAN_POINT('Ctrl Pts',(-0.170490360446879,-0.672457732793657,
2.98139101419695));
#25092=CARTESIAN_POINT('Ctrl Pts',(-0.168743555851695,-0.665206983690625,
2.99561895616294));
#25093=CARTESIAN_POINT('Ctrl Pts',(-0.166116864500515,-0.654306603263479,
3.02268687665294));
#25094=CARTESIAN_POINT('Ctrl Pts',(-0.164994936632523,-0.649652638626213,
3.03802055188041));
#25095=CARTESIAN_POINT('Ctrl Pts',(-0.163534094630633,-0.64359359422561,
3.06935267774138));
#25096=CARTESIAN_POINT('Ctrl Pts',(-0.163195228371984,-0.642188506154241,
3.08535112900039));
#25097=CARTESIAN_POINT('Ctrl Pts',(-0.163195228371985,-0.642188506154241,
3.11464887099961));
#25098=CARTESIAN_POINT('Ctrl Pts',(-0.163534094630636,-0.643593594225609,
3.13064732225863));
#25099=CARTESIAN_POINT('Ctrl Pts',(-0.164994936632528,-0.649652638626212,
3.16197944811959));
#25100=CARTESIAN_POINT('Ctrl Pts',(-0.166116864500519,-0.654306603263478,
3.17731312334706));
#25101=CARTESIAN_POINT('Ctrl Pts',(-0.168743555851701,-0.665206983690623,
3.20438104383706));
#25102=CARTESIAN_POINT('Ctrl Pts',(-0.170490360446887,-0.672457732793655,
3.21860898580305));
#25103=CARTESIAN_POINT('Ctrl Pts',(-0.17464520952695,-0.689714125571451,
3.24517174819405));
#25104=CARTESIAN_POINT('Ctrl Pts',(-0.177053154990377,-0.699719787441728,
3.2575065722869));
#25105=CARTESIAN_POINT('Ctrl Pts',(-0.180063411180705,-0.712235629767467,
3.27037878209112));
#25106=CARTESIAN_POINT('Ctrl Pts',(-0.180677622653936,-0.714789679845299,
3.27289220019637));
#25107=CARTESIAN_POINT('Ctrl Pts',(-0.181315643661017,-0.717443124828576,
3.2753817550374));
#25108=CARTESIAN_POINT('',(-0.200268840560683,-0.877435120963641,2.86185));
#25109=CARTESIAN_POINT('Origin',(-0.200268840560683,-0.877435120963641,
3.1));
#25110=CARTESIAN_POINT('Ctrl Pts',(-0.164665491127673,-0.72144665501455,
3.27639564195297));
#25111=CARTESIAN_POINT('Ctrl Pts',(-0.159249892010251,-0.722682730173014,
3.27639564195297));
#25112=CARTESIAN_POINT('Ctrl Pts',(-0.153627439993718,-0.723900860216855,
3.27607258736419));
#25113=CARTESIAN_POINT('Ctrl Pts',(-0.147927155402543,-0.725063829393324,
3.2753817550374));
#25114=CARTESIAN_POINT('',(-0.200268840560683,-0.877435120963641,3.33815));
#25115=CARTESIAN_POINT('Origin',(-0.200268840560683,-0.877435120963641,
3.1));
#25116=CARTESIAN_POINT('Ctrl Pts',(-0.255808886330153,-1.0286699245504,
3.2753817550374));
#25117=CARTESIAN_POINT('Ctrl Pts',(-0.256441802889327,-1.03132435481591,
3.27289236009202));
#25118=CARTESIAN_POINT('Ctrl Pts',(-0.257050967245519,-1.03387938890926,
3.27037910645452));
#25119=CARTESIAN_POINT('Ctrl Pts',(-0.260036088454,-1.04640086511301,3.25750707214144));
#25120=CARTESIAN_POINT('Ctrl Pts',(-0.262421852995025,-1.05641163134326,
3.24517226455888));
#25121=CARTESIAN_POINT('Ctrl Pts',(-0.266535646972229,-1.07367745534592,
3.21860957458692));
#25122=CARTESIAN_POINT('Ctrl Pts',(-0.268263728412826,-1.08093249774324,
3.2043816902577));
#25123=CARTESIAN_POINT('Ctrl Pts',(-0.270861407310783,-1.09183962883285,
3.17731372034463));
#25124=CARTESIAN_POINT('Ctrl Pts',(-0.271970325972461,-1.09649664382985,
3.16197991083841));
#25125=CARTESIAN_POINT('Ctrl Pts',(-0.273413966562287,-1.1025597136748,
3.13064753590579));
#25126=CARTESIAN_POINT('Ctrl Pts',(-0.273748708187842,-1.10396576249696,
3.11464897022091));
#25127=CARTESIAN_POINT('Ctrl Pts',(-0.273748708187841,-1.10396576249696,
3.1));
#25128=CARTESIAN_POINT('Ctrl Pts',(-0.273748708187841,-1.10396576249696,
3.08535102977909));
#25129=CARTESIAN_POINT('Ctrl Pts',(-0.273413966562285,-1.10255971367481,
3.06935246409421));
#25130=CARTESIAN_POINT('Ctrl Pts',(-0.271970325972456,-1.09649664382985,
3.03802008916159));
#25131=CARTESIAN_POINT('Ctrl Pts',(-0.270861407310774,-1.09183962883285,
3.02268627965537));
#25132=CARTESIAN_POINT('Ctrl Pts',(-0.268263728412815,-1.08093249774325,
2.9956183097423));
#25133=CARTESIAN_POINT('Ctrl Pts',(-0.266535646972218,-1.07367745534592,
2.98139042541308));
#25134=CARTESIAN_POINT('Ctrl Pts',(-0.262421852995011,-1.05641163134326,
2.95482773544112));
#25135=CARTESIAN_POINT('Ctrl Pts',(-0.260036088453991,-1.04640086511301,
2.94249292785856));
#25136=CARTESIAN_POINT('Ctrl Pts',(-0.257050967245501,-1.03387938890923,
2.92962089354545));
#25137=CARTESIAN_POINT('Ctrl Pts',(-0.256441802889302,-1.03132435481589,
2.92710763990796));
#25138=CARTESIAN_POINT('Ctrl Pts',(-0.255808886330133,-1.02866992455041,
2.9246182449626));
#25139=CARTESIAN_POINT('Origin',(0.,0.,3.1));
#25140=CARTESIAN_POINT('Ctrl Pts',(-0.945956189565651,-0.47829581581113,
2.9246182449626));
#25141=CARTESIAN_POINT('Ctrl Pts',(-0.94840323053857,-0.479503530132554,
2.92710763990799));
#25142=CARTESIAN_POINT('Ctrl Pts',(-0.950758652771283,-0.480665970039254,
2.92962089354548));
#25143=CARTESIAN_POINT('Ctrl Pts',(-0.962301937464754,-0.486362538606019,
2.94249292785856));
#25144=CARTESIAN_POINT('Ctrl Pts',(-0.971530830331082,-0.490916092100134,
2.95482773544112));
#25145=CARTESIAN_POINT('Ctrl Pts',(-0.98744835880018,-0.498768751956074,
2.98139042541308));
#25146=CARTESIAN_POINT('Ctrl Pts',(-0.994136967841286,-0.502067905597172,
2.9956183097423));
#25147=CARTESIAN_POINT('Ctrl Pts',(-1.00419259644788,-0.50702752025852,
3.02268627965537));
#25148=CARTESIAN_POINT('Ctrl Pts',(-1.00848609273962,-0.509144919340721,
3.03802008916159));
#25149=CARTESIAN_POINT('Ctrl Pts',(-1.01407590851263,-0.511901524811445,
3.06935246409421));
#25150=CARTESIAN_POINT('Ctrl Pts',(-1.01537221773608,-0.512540749062661,
3.08535102977909));
#25151=CARTESIAN_POINT('Ctrl Pts',(-1.01537221773608,-0.512540749062661,
3.1));
#25152=CARTESIAN_POINT('Ctrl Pts',(-1.01537221773608,-0.512540749062661,
3.11464897022091));
#25153=CARTESIAN_POINT('Ctrl Pts',(-1.01407590851263,-0.511901524811445,
3.13064753590579));
#25154=CARTESIAN_POINT('Ctrl Pts',(-1.00848609273962,-0.509144919340721,
3.16197991083841));
#25155=CARTESIAN_POINT('Ctrl Pts',(-1.00419259644788,-0.50702752025852,
3.17731372034463));
#25156=CARTESIAN_POINT('Ctrl Pts',(-0.994136967841286,-0.502067905597172,
3.2043816902577));
#25157=CARTESIAN_POINT('Ctrl Pts',(-0.98744835880018,-0.498768751956074,
3.21860957458692));
#25158=CARTESIAN_POINT('Ctrl Pts',(-0.971530830331082,-0.490916092100134,
3.24517226455888));
#25159=CARTESIAN_POINT('Ctrl Pts',(-0.962301937464754,-0.486362538606019,
3.25750707214144));
#25160=CARTESIAN_POINT('Ctrl Pts',(-0.950758652771256,-0.480665970039241,
3.27037910645455));
#25161=CARTESIAN_POINT('Ctrl Pts',(-0.948403230538551,-0.479503530132544,
3.27289236009204));
#25162=CARTESIAN_POINT('Ctrl Pts',(-0.945956189565651,-0.47829581581113,
3.2753817550374));
#25163=CARTESIAN_POINT('Origin',(0.,0.,3.1));
#25164=CARTESIAN_POINT('',(-0.659108801429989,-0.336415796117726,3.2753817550374));
#25165=CARTESIAN_POINT('Origin',(0.,0.,3.2753817550374));
#25166=CARTESIAN_POINT('Ctrl Pts',(-0.659108801429989,-0.336415796117726,
3.2753817550374));
#25167=CARTESIAN_POINT('Ctrl Pts',(-0.656663856882733,-0.335203324573485,
3.27289220019637));
#25168=CARTESIAN_POINT('Ctrl Pts',(-0.654310517083416,-0.334036183055557,
3.27037878209112));
#25169=CARTESIAN_POINT('Ctrl Pts',(-0.642778318074505,-0.328316363349215,
3.2575065722869));
#25170=CARTESIAN_POINT('Ctrl Pts',(-0.633559337310756,-0.323742320881684,
3.24517174819405));
#25171=CARTESIAN_POINT('Ctrl Pts',(-0.617660139225852,-0.315851733904997,
3.21860898580305));
#25172=CARTESIAN_POINT('Ctrl Pts',(-0.610979882131038,-0.312535281885735,
3.20438104383706));
#25173=CARTESIAN_POINT('Ctrl Pts',(-0.600937290811893,-0.307548884337655,
3.17731312334706));
#25174=CARTESIAN_POINT('Ctrl Pts',(-0.596649663221733,-0.305419480986011,
3.16197944811959));
#25175=CARTESIAN_POINT('Ctrl Pts',(-0.591067599641059,-0.302647001124175,
3.13064732225863));
#25176=CARTESIAN_POINT('Ctrl Pts',(-0.589773144897572,-0.302003969440185,
3.11464887099961));
#25177=CARTESIAN_POINT('Ctrl Pts',(-0.589773144897572,-0.302003969440185,
3.08535112900039));
#25178=CARTESIAN_POINT('Ctrl Pts',(-0.591067599641059,-0.302647001124175,
3.06935267774138));
#25179=CARTESIAN_POINT('Ctrl Pts',(-0.596649663221733,-0.305419480986011,
3.03802055188041));
#25180=CARTESIAN_POINT('Ctrl Pts',(-0.600937290811893,-0.307548884337655,
3.02268687665294));
#25181=CARTESIAN_POINT('Ctrl Pts',(-0.610979882131038,-0.312535281885735,
2.99561895616294));
#25182=CARTESIAN_POINT('Ctrl Pts',(-0.617660139225853,-0.315851733904994,
2.98139101419695));
#25183=CARTESIAN_POINT('Ctrl Pts',(-0.633559337310756,-0.323742320881681,
2.95482825180595));
#25184=CARTESIAN_POINT('Ctrl Pts',(-0.642778318074504,-0.328316363349218,
2.9424934277131));
#25185=CARTESIAN_POINT('Ctrl Pts',(-0.654310517083415,-0.33403618305556,
2.92962121790888));
#25186=CARTESIAN_POINT('Ctrl Pts',(-0.656663856882733,-0.335203324573485,
2.92710779980363));
#25187=CARTESIAN_POINT('Ctrl Pts',(-0.659108801429989,-0.336415796117726,
2.9246182449626));
#25188=CARTESIAN_POINT('Origin',(-0.810871981112177,-0.390495365205802,
3.1));
#25189=CARTESIAN_POINT('',(-0.673968076611316,-0.305560193266145,3.2753817550374));
#25190=CARTESIAN_POINT('',(-0.66671696224779,-0.321073966946993,3.27639564195297));
#25191=CARTESIAN_POINT('Ctrl Pts',(-0.673968076611316,-0.305560193266145,
3.2753817550374));
#25192=CARTESIAN_POINT('Ctrl Pts',(-0.671565832849124,-0.310858774834149,
3.27607258736419));
#25193=CARTESIAN_POINT('Ctrl Pts',(-0.669127130594873,-0.316069200804934,
3.27639564195297));
#25194=CARTESIAN_POINT('Ctrl Pts',(-0.66671696224779,-0.321073966946993,
3.27639564195297));
#25195=CARTESIAN_POINT('Ctrl Pts',(-0.673968076611316,-0.305560193266145,
2.9246182449626));
#25196=CARTESIAN_POINT('Ctrl Pts',(-0.671495730195107,-0.30440462228909,
2.92710779980363));
#25197=CARTESIAN_POINT('Ctrl Pts',(-0.669115938846714,-0.303292407978791,
2.92962121790888));
#25198=CARTESIAN_POINT('Ctrl Pts',(-0.657453795251194,-0.297842420986912,
2.9424934277131));
#25199=CARTESIAN_POINT('Ctrl Pts',(-0.6481297243582,-0.293486600421324,
2.95482825180595));
#25200=CARTESIAN_POINT('Ctrl Pts',(-0.632047627181004,-0.285975807323195,
2.98139101419695));
#25201=CARTESIAN_POINT('Ctrl Pts',(-0.625289648409841,-0.282820746027851,
2.99561895616294));
#25202=CARTESIAN_POINT('Ctrl Pts',(-0.615129672550929,-0.278078099988225,
3.02268687665294));
#25203=CARTESIAN_POINT('Ctrl Pts',(-0.610791545895107,-0.276053559026934,
3.03802055188041));
#25204=CARTESIAN_POINT('Ctrl Pts',(-0.605143574138738,-0.273417938902139,
3.06935267774138));
#25205=CARTESIAN_POINT('Ctrl Pts',(-0.603833752392438,-0.272806817128289,
3.08535112900039));
#25206=CARTESIAN_POINT('Ctrl Pts',(-0.603833752392438,-0.272806817128289,
3.11464887099961));
#25207=CARTESIAN_POINT('Ctrl Pts',(-0.605143574138739,-0.273417938902138,
3.13064732225863));
#25208=CARTESIAN_POINT('Ctrl Pts',(-0.610791545895107,-0.276053559026933,
3.16197944811959));
#25209=CARTESIAN_POINT('Ctrl Pts',(-0.615129672550929,-0.278078099988225,
3.17731312334706));
#25210=CARTESIAN_POINT('Ctrl Pts',(-0.625289648409841,-0.282820746027851,
3.20438104383706));
#25211=CARTESIAN_POINT('Ctrl Pts',(-0.632047627181007,-0.285975807323192,
3.21860898580305));
#25212=CARTESIAN_POINT('Ctrl Pts',(-0.648129724358202,-0.293486600421321,
3.24517174819405));
#25213=CARTESIAN_POINT('Ctrl Pts',(-0.657453795251192,-0.297842420986915,
3.2575065722869));
#25214=CARTESIAN_POINT('Ctrl Pts',(-0.669115938846713,-0.303292407978794,
3.27037878209112));
#25215=CARTESIAN_POINT('Ctrl Pts',(-0.671495730195106,-0.30440462228909,
3.27289220019637));
#25216=CARTESIAN_POINT('Ctrl Pts',(-0.673968076611316,-0.305560193266145,
3.2753817550374));
#25217=CARTESIAN_POINT('',(-0.810871981112177,-0.390495365205802,2.86185));
#25218=CARTESIAN_POINT('Origin',(-0.810871981112177,-0.390495365205802,
3.1));
#25219=CARTESIAN_POINT('Ctrl Pts',(-0.66671696224779,-0.321073966946993,
3.27639564195297));
#25220=CARTESIAN_POINT('Ctrl Pts',(-0.664306793900707,-0.326078733089052,
3.27639564195297));
#25221=CARTESIAN_POINT('Ctrl Pts',(-0.661753624824974,-0.331234034743915,
3.27607258736419));
#25222=CARTESIAN_POINT('Ctrl Pts',(-0.659108801429989,-0.336415796117726,
3.2753817550374));
#25223=CARTESIAN_POINT('',(-0.810871981112177,-0.390495365205802,3.33815));
#25224=CARTESIAN_POINT('Origin',(-0.810871981112177,-0.390495365205802,
3.1));
#25225=CARTESIAN_POINT('Ctrl Pts',(-0.963740763933202,-0.441365766607978,
3.2753817550374));
#25226=CARTESIAN_POINT('Ctrl Pts',(-0.966210698102864,-0.442525942716529,
3.27289236009202));
#25227=CARTESIAN_POINT('Ctrl Pts',(-0.968588111959567,-0.443642716545468,
3.27037910645452));
#25228=CARTESIAN_POINT('Ctrl Pts',(-0.980238988893433,-0.449115867522948,
3.25750707214144));
#25229=CARTESIAN_POINT('Ctrl Pts',(-0.989553220956837,-0.453492212348372,
3.24517226455888));
#25230=CARTESIAN_POINT('Ctrl Pts',(-1.0056170943246,-0.461040983890949,
3.21860957458692));
#25231=CARTESIAN_POINT('Ctrl Pts',(-1.01236675603246,-0.464213360363215,
3.2043816902577));
#25232=CARTESIAN_POINT('Ctrl Pts',(-1.0225139208031,-0.468982898221355,
3.17731372034463));
#25233=CARTESIAN_POINT('Ctrl Pts',(-1.02684632121873,-0.471019512057877,
3.16197991083841));
#25234=CARTESIAN_POINT('Ctrl Pts',(-1.03248671528923,-0.473671090611669,
3.13064753590579));
#25235=CARTESIAN_POINT('Ctrl Pts',(-1.03379471651407,-0.474286036171845,
3.11464897022091));
#25236=CARTESIAN_POINT('Ctrl Pts',(-1.03379471651407,-0.474286036171845,
3.1));
#25237=CARTESIAN_POINT('Ctrl Pts',(-1.03379471651407,-0.474286036171845,
3.08535102977909));
#25238=CARTESIAN_POINT('Ctrl Pts',(-1.03248671528923,-0.473671090611669,
3.06935246409421));
#25239=CARTESIAN_POINT('Ctrl Pts',(-1.02684632121873,-0.471019512057877,
3.03802008916159));
#25240=CARTESIAN_POINT('Ctrl Pts',(-1.0225139208031,-0.468982898221355,
3.02268627965537));
#25241=CARTESIAN_POINT('Ctrl Pts',(-1.01236675603246,-0.464213360363215,
2.9956183097423));
#25242=CARTESIAN_POINT('Ctrl Pts',(-1.0056170943246,-0.461040983890949,
2.98139042541308));
#25243=CARTESIAN_POINT('Ctrl Pts',(-0.989553220956837,-0.453492212348372,
2.95482773544112));
#25244=CARTESIAN_POINT('Ctrl Pts',(-0.980238988893433,-0.449115867522948,
2.94249292785856));
#25245=CARTESIAN_POINT('Ctrl Pts',(-0.96858811195954,-0.443642716545455,
2.92962089354545));
#25246=CARTESIAN_POINT('Ctrl Pts',(-0.966210698102844,-0.44252594271652,
2.92710763990797));
#25247=CARTESIAN_POINT('Ctrl Pts',(-0.963740763933202,-0.441365766607979,
2.9246182449626));
#25248=CARTESIAN_POINT('Origin',(0.,0.,3.1));
#25249=CARTESIAN_POINT('Ctrl Pts',(-0.963740763933198,0.441365766607986,
2.9246182449626));
#25250=CARTESIAN_POINT('Ctrl Pts',(-0.96621069810286,0.442525942716537,
2.92710763990798));
#25251=CARTESIAN_POINT('Ctrl Pts',(-0.968588111959567,0.443642716545468,
2.92962089354548));
#25252=CARTESIAN_POINT('Ctrl Pts',(-0.980238988893433,0.449115867522948,
2.94249292785856));
#25253=CARTESIAN_POINT('Ctrl Pts',(-0.989553220956834,0.453492212348377,
2.95482773544112));
#25254=CARTESIAN_POINT('Ctrl Pts',(-1.0056170943246,0.461040983890953,2.98139042541308));
#25255=CARTESIAN_POINT('Ctrl Pts',(-1.01236675603246,0.464213360363211,
2.9956183097423));
#25256=CARTESIAN_POINT('Ctrl Pts',(-1.02251392080311,0.468982898221349,
3.02268627965537));
#25257=CARTESIAN_POINT('Ctrl Pts',(-1.02684632121873,0.471019512057878,
3.03802008916159));
#25258=CARTESIAN_POINT('Ctrl Pts',(-1.03248671528923,0.473671090611668,
3.06935246409421));
#25259=CARTESIAN_POINT('Ctrl Pts',(-1.03379471651406,0.474286036171856,
3.08535102977909));
#25260=CARTESIAN_POINT('Ctrl Pts',(-1.03379471651406,0.474286036171855,
3.1));
#25261=CARTESIAN_POINT('Ctrl Pts',(-1.03379471651406,0.474286036171854,
3.11464897022091));
#25262=CARTESIAN_POINT('Ctrl Pts',(-1.03248671528923,0.473671090611665,
3.13064753590579));
#25263=CARTESIAN_POINT('Ctrl Pts',(-1.02684632121874,0.471019512057872,
3.16197991083841));
#25264=CARTESIAN_POINT('Ctrl Pts',(-1.02251392080311,0.468982898221341,
3.17731372034463));
#25265=CARTESIAN_POINT('Ctrl Pts',(-1.01236675603247,0.4642133603632,3.2043816902577));
#25266=CARTESIAN_POINT('Ctrl Pts',(-1.00561709432461,0.461040983890937,
3.21860957458692));
#25267=CARTESIAN_POINT('Ctrl Pts',(-0.989553220956842,0.453492212348359,
3.24517226455888));
#25268=CARTESIAN_POINT('Ctrl Pts',(-0.980238988893438,0.449115867522939,
3.25750707214144));
#25269=CARTESIAN_POINT('Ctrl Pts',(-0.968588111959544,0.443642716545446,
3.27037910645455));
#25270=CARTESIAN_POINT('Ctrl Pts',(-0.966210698102848,0.442525942716513,
3.27289236009203));
#25271=CARTESIAN_POINT('Ctrl Pts',(-0.963740763933205,0.441365766607971,
3.2753817550374));
#25272=CARTESIAN_POINT('Origin',(0.,0.,3.1));
#25273=CARTESIAN_POINT('',(-0.74,-9.06238631369041E-17,3.2753817550374));
#25274=CARTESIAN_POINT('Origin',(0.,0.,3.2753817550374));
#25275=CARTESIAN_POINT('',(-0.673968076611317,0.305560193266142,3.2753817550374));
#25276=CARTESIAN_POINT('Origin',(0.,0.,3.2753817550374));
#25277=CARTESIAN_POINT('Ctrl Pts',(-0.673968076611317,0.305560193266142,
3.2753817550374));
#25278=CARTESIAN_POINT('Ctrl Pts',(-0.671495730195108,0.304404622289088,
3.27289220019637));
#25279=CARTESIAN_POINT('Ctrl Pts',(-0.669115938846715,0.303292407978788,
3.27037878209112));
#25280=CARTESIAN_POINT('Ctrl Pts',(-0.657453795251195,0.29784242098691,
3.2575065722869));
#25281=CARTESIAN_POINT('Ctrl Pts',(-0.648129724358203,0.293486600421318,
3.24517174819405));
#25282=CARTESIAN_POINT('Ctrl Pts',(-0.632047627181007,0.28597580732319,
3.21860898580305));
#25283=CARTESIAN_POINT('Ctrl Pts',(-0.625289648409841,0.282820746027851,
3.20438104383706));
#25284=CARTESIAN_POINT('Ctrl Pts',(-0.615129672550928,0.278078099988226,
3.17731312334706));
#25285=CARTESIAN_POINT('Ctrl Pts',(-0.610791545895108,0.276053559026932,
3.16197944811959));
#25286=CARTESIAN_POINT('Ctrl Pts',(-0.605143574138739,0.273417938902138,
3.13064732225863));
#25287=CARTESIAN_POINT('Ctrl Pts',(-0.603833752392439,0.272806817128288,
3.11464887099961));
#25288=CARTESIAN_POINT('Ctrl Pts',(-0.603833752392438,0.272806817128289,
3.08535112900039));
#25289=CARTESIAN_POINT('Ctrl Pts',(-0.605143574138737,0.273417938902141,
3.06935267774137));
#25290=CARTESIAN_POINT('Ctrl Pts',(-0.610791545895105,0.276053559026937,
3.03802055188041));
#25291=CARTESIAN_POINT('Ctrl Pts',(-0.615129672550927,0.278078099988229,
3.02268687665294));
#25292=CARTESIAN_POINT('Ctrl Pts',(-0.625289648409839,0.282820746027856,
2.99561895616294));
#25293=CARTESIAN_POINT('Ctrl Pts',(-0.632047627181002,0.285975807323201,
2.98139101419695));
#25294=CARTESIAN_POINT('Ctrl Pts',(-0.648129724358197,0.293486600421331,
2.95482825180595));
#25295=CARTESIAN_POINT('Ctrl Pts',(-0.65745379525119,0.297842420986921,
2.9424934277131));
#25296=CARTESIAN_POINT('Ctrl Pts',(-0.66911593884671,0.3032924079788,2.92962121790888));
#25297=CARTESIAN_POINT('Ctrl Pts',(-0.671495730195102,0.304404622289099,
2.92710779980363));
#25298=CARTESIAN_POINT('Ctrl Pts',(-0.673968076611311,0.305560193266154,
2.9246182449626));
#25299=CARTESIAN_POINT('Origin',(-0.810871981112177,0.390495365205802,3.1));
#25300=CARTESIAN_POINT('',(-0.659108801429987,0.336415796117729,3.2753817550374));
#25301=CARTESIAN_POINT('',(-0.66671696224779,0.321073966946993,3.27639564195297));
#25302=CARTESIAN_POINT('Ctrl Pts',(-0.659108801429987,0.336415796117729,
3.2753817550374));
#25303=CARTESIAN_POINT('Ctrl Pts',(-0.661753624824973,0.331234034743917,
3.27607258736419));
#25304=CARTESIAN_POINT('Ctrl Pts',(-0.664306793900707,0.326078733089053,
3.27639564195297));
#25305=CARTESIAN_POINT('Ctrl Pts',(-0.66671696224779,0.321073966946993,
3.27639564195297));
#25306=CARTESIAN_POINT('Ctrl Pts',(-0.659108801429993,0.336415796117718,
2.9246182449626));
#25307=CARTESIAN_POINT('Ctrl Pts',(-0.656663856882737,0.335203324573476,
2.92710779980363));
#25308=CARTESIAN_POINT('Ctrl Pts',(-0.654310517083419,0.334036183055551,
2.92962121790888));
#25309=CARTESIAN_POINT('Ctrl Pts',(-0.642778318074508,0.32831636334921,
2.9424934277131));
#25310=CARTESIAN_POINT('Ctrl Pts',(-0.633559337310759,0.323742320881676,
2.95482825180595));
#25311=CARTESIAN_POINT('Ctrl Pts',(-0.617660139225855,0.31585173390499,
2.98139101419695));
#25312=CARTESIAN_POINT('Ctrl Pts',(-0.61097988213104,0.31253528188573,2.99561895616294));
#25313=CARTESIAN_POINT('Ctrl Pts',(-0.600937290811895,0.307548884337651,
3.02268687665294));
#25314=CARTESIAN_POINT('Ctrl Pts',(-0.596649663221735,0.305419480986006,
3.03802055188041));
#25315=CARTESIAN_POINT('Ctrl Pts',(-0.591067599641061,0.302647001124171,
3.06935267774138));
#25316=CARTESIAN_POINT('Ctrl Pts',(-0.589773144897572,0.302003969440184,
3.08535112900039));
#25317=CARTESIAN_POINT('Ctrl Pts',(-0.589773144897571,0.302003969440185,
3.11464887099961));
#25318=CARTESIAN_POINT('Ctrl Pts',(-0.591067599641059,0.302647001124175,
3.13064732225862));
#25319=CARTESIAN_POINT('Ctrl Pts',(-0.596649663221732,0.305419480986012,
3.16197944811959));
#25320=CARTESIAN_POINT('Ctrl Pts',(-0.600937290811894,0.307548884337654,
3.17731312334706));
#25321=CARTESIAN_POINT('Ctrl Pts',(-0.610979882131038,0.312535281885736,
3.20438104383706));
#25322=CARTESIAN_POINT('Ctrl Pts',(-0.61766013922585,0.315851733905002,
3.21860898580305));
#25323=CARTESIAN_POINT('Ctrl Pts',(-0.633559337310753,0.32374232088169,
3.24517174819405));
#25324=CARTESIAN_POINT('Ctrl Pts',(-0.642778318074502,0.32831636334922,
3.2575065722869));
#25325=CARTESIAN_POINT('Ctrl Pts',(-0.654310517083413,0.334036183055563,
3.27037878209112));
#25326=CARTESIAN_POINT('Ctrl Pts',(-0.656663856882731,0.335203324573488,
3.27289220019637));
#25327=CARTESIAN_POINT('Ctrl Pts',(-0.659108801429987,0.336415796117729,
3.2753817550374));
#25328=CARTESIAN_POINT('',(-0.810871981112177,0.390495365205802,2.86185));
#25329=CARTESIAN_POINT('Origin',(-0.810871981112177,0.390495365205802,3.1));
#25330=CARTESIAN_POINT('Ctrl Pts',(-0.66671696224779,0.321073966946993,
3.27639564195297));
#25331=CARTESIAN_POINT('Ctrl Pts',(-0.669127130594873,0.316069200804933,
3.27639564195297));
#25332=CARTESIAN_POINT('Ctrl Pts',(-0.671565832849125,0.310858774834148,
3.27607258736419));
#25333=CARTESIAN_POINT('Ctrl Pts',(-0.673968076611317,0.305560193266142,
3.2753817550374));
#25334=CARTESIAN_POINT('',(-0.810871981112177,0.390495365205802,3.33815));
#25335=CARTESIAN_POINT('Origin',(-0.810871981112177,0.390495365205802,3.1));
#25336=CARTESIAN_POINT('Ctrl Pts',(-0.945956189565646,0.47829581581114,
3.2753817550374));
#25337=CARTESIAN_POINT('Ctrl Pts',(-0.948403230538565,0.479503530132563,
3.27289236009202));
#25338=CARTESIAN_POINT('Ctrl Pts',(-0.950758652771278,0.480665970039264,
3.27037910645452));
#25339=CARTESIAN_POINT('Ctrl Pts',(-0.962301937464749,0.486362538606029,
3.25750707214144));
#25340=CARTESIAN_POINT('Ctrl Pts',(-0.971530830331079,0.490916092100141,
3.24517226455888));
#25341=CARTESIAN_POINT('Ctrl Pts',(-0.987448358800177,0.49876875195608,
3.21860957458692));
#25342=CARTESIAN_POINT('Ctrl Pts',(-0.994136967841278,0.502067905597186,
3.2043816902577));
#25343=CARTESIAN_POINT('Ctrl Pts',(-1.00419259644787,0.507027520258534,
3.17731372034463));
#25344=CARTESIAN_POINT('Ctrl Pts',(-1.00848609273961,0.509144919340726,
3.16197991083841));
#25345=CARTESIAN_POINT('Ctrl Pts',(-1.01407590851262,0.511901524811448,
3.13064753590579));
#25346=CARTESIAN_POINT('Ctrl Pts',(-1.01537221773608,0.512540749062652,
3.11464897022091));
#25347=CARTESIAN_POINT('Ctrl Pts',(-1.01537221773608,0.512540749062652,
3.1));
#25348=CARTESIAN_POINT('Ctrl Pts',(-1.01537221773609,0.512540749062651,
3.08535102977909));
#25349=CARTESIAN_POINT('Ctrl Pts',(-1.01407590851262,0.511901524811446,
3.06935246409421));
#25350=CARTESIAN_POINT('Ctrl Pts',(-1.00848609273962,0.509144919340721,
3.03802008916159));
#25351=CARTESIAN_POINT('Ctrl Pts',(-1.00419259644788,0.507027520258526,
3.02268627965537));
#25352=CARTESIAN_POINT('Ctrl Pts',(-0.994136967841284,0.502067905597176,
2.9956183097423));
#25353=CARTESIAN_POINT('Ctrl Pts',(-0.987448358800183,0.498768751956068,
2.98139042541308));
#25354=CARTESIAN_POINT('Ctrl Pts',(-0.971530830331086,0.490916092100127,
2.95482773544112));
#25355=CARTESIAN_POINT('Ctrl Pts',(-0.962301937464754,0.48636253860602,
2.94249292785856));
#25356=CARTESIAN_POINT('Ctrl Pts',(-0.950758652771256,0.480665970039241,
2.92962089354545));
#25357=CARTESIAN_POINT('Ctrl Pts',(-0.948403230538554,0.479503530132536,
2.92710763990796));
#25358=CARTESIAN_POINT('Ctrl Pts',(-0.945956189565655,0.478295815811122,
2.9246182449626));
#25359=CARTESIAN_POINT('Origin',(0.,0.,3.1));
#25360=CARTESIAN_POINT('Ctrl Pts',(-0.255808886330142,1.0286699245504,2.9246182449626));
#25361=CARTESIAN_POINT('Ctrl Pts',(-0.256441802889316,1.03132435481591,
2.92710763990798));
#25362=CARTESIAN_POINT('Ctrl Pts',(-0.257050967245508,1.03387938890926,
2.92962089354548));
#25363=CARTESIAN_POINT('Ctrl Pts',(-0.26003608845399,1.04640086511301,2.94249292785856));
#25364=CARTESIAN_POINT('Ctrl Pts',(-0.262421852995016,1.05641163134326,
2.95482773544112));
#25365=CARTESIAN_POINT('Ctrl Pts',(-0.266535646972222,1.07367745534592,
2.98139042541308));
#25366=CARTESIAN_POINT('Ctrl Pts',(-0.26826372841281,1.08093249774325,2.9956183097423));
#25367=CARTESIAN_POINT('Ctrl Pts',(-0.270861407310768,1.09183962883285,
3.02268627965537));
#25368=CARTESIAN_POINT('Ctrl Pts',(-0.271970325972459,1.09649664382985,
3.03802008916159));
#25369=CARTESIAN_POINT('Ctrl Pts',(-0.273413966562286,1.1025597136748,3.06935246409421));
#25370=CARTESIAN_POINT('Ctrl Pts',(-0.273748708187841,1.10396576249696,
3.08535102977909));
#25371=CARTESIAN_POINT('Ctrl Pts',(-0.273748708187841,1.10396576249696,
3.1));
#25372=CARTESIAN_POINT('Ctrl Pts',(-0.273748708187841,1.10396576249696,
3.11464897022091));
#25373=CARTESIAN_POINT('Ctrl Pts',(-0.273413966562286,1.1025597136748,3.13064753590579));
#25374=CARTESIAN_POINT('Ctrl Pts',(-0.271970325972459,1.09649664382985,
3.16197991083841));
#25375=CARTESIAN_POINT('Ctrl Pts',(-0.270861407310768,1.09183962883285,
3.17731372034463));
#25376=CARTESIAN_POINT('Ctrl Pts',(-0.26826372841281,1.08093249774325,3.2043816902577));
#25377=CARTESIAN_POINT('Ctrl Pts',(-0.266535646972222,1.07367745534592,
3.21860957458692));
#25378=CARTESIAN_POINT('Ctrl Pts',(-0.262421852995016,1.05641163134326,
3.24517226455888));
#25379=CARTESIAN_POINT('Ctrl Pts',(-0.26003608845399,1.04640086511301,3.25750707214144));
#25380=CARTESIAN_POINT('Ctrl Pts',(-0.257050967245501,1.03387938890923,
3.27037910645455));
#25381=CARTESIAN_POINT('Ctrl Pts',(-0.256441802889309,1.03132435481589,
3.27289236009204));
#25382=CARTESIAN_POINT('Ctrl Pts',(-0.25580888633014,1.0286699245504,3.2753817550374));
#25383=CARTESIAN_POINT('Origin',(0.,0.,3.1));
#25384=CARTESIAN_POINT('',(-0.181315643661013,0.717443124828577,3.2753817550374));
#25385=CARTESIAN_POINT('Origin',(0.,0.,3.2753817550374));
#25386=CARTESIAN_POINT('Ctrl Pts',(-0.181315643661013,0.717443124828577,
3.2753817550374));
#25387=CARTESIAN_POINT('Ctrl Pts',(-0.180677622653932,0.7147896798453,3.27289220019637));
#25388=CARTESIAN_POINT('Ctrl Pts',(-0.180063411180699,0.712235629767469,
3.27037878209112));
#25389=CARTESIAN_POINT('Ctrl Pts',(-0.177053154990371,0.699719787441729,
3.2575065722869));
#25390=CARTESIAN_POINT('Ctrl Pts',(-0.174645209526945,0.689714125571452,
3.24517174819405));
#25391=CARTESIAN_POINT('Ctrl Pts',(-0.170490360446883,0.672457732793656,
3.21860898580305));
#25392=CARTESIAN_POINT('Ctrl Pts',(-0.1687435558517,0.665206983690623,3.20438104383706));
#25393=CARTESIAN_POINT('Ctrl Pts',(-0.166116864500519,0.654306603263478,
3.17731312334706));
#25394=CARTESIAN_POINT('Ctrl Pts',(-0.164994936632528,0.649652638626212,
3.16197944811959));
#25395=CARTESIAN_POINT('Ctrl Pts',(-0.163534094630637,0.643593594225609,
3.13064732225863));
#25396=CARTESIAN_POINT('Ctrl Pts',(-0.163195228371982,0.642188506154242,
3.11464887099961));
#25397=CARTESIAN_POINT('Ctrl Pts',(-0.163195228371982,0.642188506154242,
3.08535112900039));
#25398=CARTESIAN_POINT('Ctrl Pts',(-0.163534094630636,0.643593594225609,
3.06935267774138));
#25399=CARTESIAN_POINT('Ctrl Pts',(-0.164994936632526,0.649652638626212,
3.03802055188041));
#25400=CARTESIAN_POINT('Ctrl Pts',(-0.166116864500519,0.654306603263478,
3.02268687665294));
#25401=CARTESIAN_POINT('Ctrl Pts',(-0.1687435558517,0.665206983690623,2.99561895616294));
#25402=CARTESIAN_POINT('Ctrl Pts',(-0.170490360446883,0.672457732793656,
2.98139101419695));
#25403=CARTESIAN_POINT('Ctrl Pts',(-0.174645209526944,0.689714125571452,
2.95482825180595));
#25404=CARTESIAN_POINT('Ctrl Pts',(-0.177053154990374,0.699719787441729,
2.9424934277131));
#25405=CARTESIAN_POINT('Ctrl Pts',(-0.180063411180702,0.712235629767469,
2.92962121790888));
#25406=CARTESIAN_POINT('Ctrl Pts',(-0.180677622653932,0.7147896798453,2.92710779980363));
#25407=CARTESIAN_POINT('Ctrl Pts',(-0.181315643661013,0.717443124828577,
2.9246182449626));
#25408=CARTESIAN_POINT('Origin',(-0.200268840560683,0.877435120963641,3.1));
#25409=CARTESIAN_POINT('',(-0.147927155402546,0.725063829393324,3.2753817550374));
#25410=CARTESIAN_POINT('',(-0.164665491127673,0.72144665501455,3.27639564195297));
#25411=CARTESIAN_POINT('Ctrl Pts',(-0.147927155402546,0.725063829393324,
3.2753817550374));
#25412=CARTESIAN_POINT('Ctrl Pts',(-0.15362743999372,0.723900860216854,
3.27607258736419));
#25413=CARTESIAN_POINT('Ctrl Pts',(-0.159249892010252,0.722682730173014,
3.27639564195297));
#25414=CARTESIAN_POINT('Ctrl Pts',(-0.164665491127673,0.72144665501455,
3.27639564195297));
#25415=CARTESIAN_POINT('Ctrl Pts',(-0.147927155402546,0.725063829393324,
2.9246182449626));
#25416=CARTESIAN_POINT('Ctrl Pts',(-0.147350705836107,0.722396331130512,
2.92710779980363));
#25417=CARTESIAN_POINT('Ctrl Pts',(-0.146795930454133,0.719828715152708,
2.92962121790888));
#25418=CARTESIAN_POINT('Ctrl Pts',(-0.144077657099531,0.70724622965008,
2.9424934277131));
#25419=CARTESIAN_POINT('Ctrl Pts',(-0.141905847013067,0.697186671420937,
2.95482825180595));
#25420=CARTESIAN_POINT('Ctrl Pts',(-0.138161968462924,0.679836477301521,
2.98139101419695));
#25421=CARTESIAN_POINT('Ctrl Pts',(-0.136589802889265,0.672545867981452,
2.99561895616294));
#25422=CARTESIAN_POINT('Ctrl Pts',(-0.134226872204734,0.661585285903343,
3.02268687665294));
#25423=CARTESIAN_POINT('Ctrl Pts',(-0.133218414707291,0.656905422394462,
3.03802055188041));
#25424=CARTESIAN_POINT('Ctrl Pts',(-0.131905667031906,0.65081257643024,
3.06935267774138));
#25425=CARTESIAN_POINT('Ctrl Pts',(-0.13160133011514,0.649399607261912,
3.08535112900039));
#25426=CARTESIAN_POINT('Ctrl Pts',(-0.13160133011514,0.649399607261913,
3.11464887099961));
#25427=CARTESIAN_POINT('Ctrl Pts',(-0.131905667031905,0.650812576430241,
3.13064732225863));
#25428=CARTESIAN_POINT('Ctrl Pts',(-0.13321841470729,0.656905422394463,
3.16197944811959));
#25429=CARTESIAN_POINT('Ctrl Pts',(-0.134226872204734,0.661585285903343,
3.17731312334706));
#25430=CARTESIAN_POINT('Ctrl Pts',(-0.136589802889265,0.672545867981452,
3.20438104383706));
#25431=CARTESIAN_POINT('Ctrl Pts',(-0.138161968462923,0.679836477301522,
3.21860898580305));
#25432=CARTESIAN_POINT('Ctrl Pts',(-0.141905847013066,0.697186671420939,
3.24517174819405));
#25433=CARTESIAN_POINT('Ctrl Pts',(-0.144077657099534,0.707246229650079,
3.2575065722869));
#25434=CARTESIAN_POINT('Ctrl Pts',(-0.146795930454136,0.719828715152707,
3.27037878209112));
#25435=CARTESIAN_POINT('Ctrl Pts',(-0.147350705836107,0.722396331130512,
3.27289220019637));
#25436=CARTESIAN_POINT('Ctrl Pts',(-0.147927155402546,0.725063829393324,
3.2753817550374));
#25437=CARTESIAN_POINT('',(-0.200268840560683,0.877435120963641,2.86185));
#25438=CARTESIAN_POINT('Origin',(-0.200268840560683,0.877435120963641,3.1));
#25439=CARTESIAN_POINT('Ctrl Pts',(-0.164665491127673,0.72144665501455,
3.27639564195297));
#25440=CARTESIAN_POINT('Ctrl Pts',(-0.170081090245093,0.720210579856085,
3.27639564195297));
#25441=CARTESIAN_POINT('Ctrl Pts',(-0.175675271291417,0.7188685865987,3.27607258736419));
#25442=CARTESIAN_POINT('Ctrl Pts',(-0.181315643661013,0.717443124828577,
3.2753817550374));
#25443=CARTESIAN_POINT('',(-0.200268840560683,0.877435120963641,3.33815));
#25444=CARTESIAN_POINT('Origin',(-0.200268840560683,0.877435120963641,3.1));
#25445=CARTESIAN_POINT('Ctrl Pts',(-0.215847310465459,1.03779089346786,
3.2753817550374));
#25446=CARTESIAN_POINT('Ctrl Pts',(-0.216428786478488,1.04045706470235,
3.27289236009202));
#25447=CARTESIAN_POINT('Ctrl Pts',(-0.21698853610412,1.04302337738549,3.27037910645452));
#25448=CARTESIAN_POINT('Ctrl Pts',(-0.219731899742916,1.0556000331769,3.25750707214144));
#25449=CARTESIAN_POINT('Ctrl Pts',(-0.221925908848716,1.06565456633392,
3.24517226455888));
#25450=CARTESIAN_POINT('Ctrl Pts',(-0.225710868823508,1.08299544455179,
3.21860957458692));
#25451=CARTESIAN_POINT('Ctrl Pts',(-0.22730176616715,1.09028179832403,3.2043816902577));
#25452=CARTESIAN_POINT('Ctrl Pts',(-0.229693765171487,1.10123587450717,
3.17731372034463));
#25453=CARTESIAN_POINT('Ctrl Pts',(-0.230715267060289,1.10591284181213,
3.16197991083841));
#25454=CARTESIAN_POINT('Ctrl Pts',(-0.232045259247275,1.11200185116341,
3.13064753590579));
#25455=CARTESIAN_POINT('Ctrl Pts',(-0.232353729184197,1.11341389632706,
3.11464897022091));
#25456=CARTESIAN_POINT('Ctrl Pts',(-0.232353729184197,1.11341389632706,
3.1));
#25457=CARTESIAN_POINT('Ctrl Pts',(-0.232353729184197,1.11341389632706,
3.08535102977909));
#25458=CARTESIAN_POINT('Ctrl Pts',(-0.232045259247275,1.11200185116341,
3.06935246409421));
#25459=CARTESIAN_POINT('Ctrl Pts',(-0.230715267060289,1.10591284181213,
3.03802008916159));
#25460=CARTESIAN_POINT('Ctrl Pts',(-0.229693765171487,1.10123587450717,
3.02268627965537));
#25461=CARTESIAN_POINT('Ctrl Pts',(-0.22730176616715,1.09028179832403,2.9956183097423));
#25462=CARTESIAN_POINT('Ctrl Pts',(-0.225710868823508,1.08299544455179,
2.98139042541308));
#25463=CARTESIAN_POINT('Ctrl Pts',(-0.221925908848717,1.06565456633392,
2.95482773544113));
#25464=CARTESIAN_POINT('Ctrl Pts',(-0.219731899742916,1.0556000331769,2.94249292785856));
#25465=CARTESIAN_POINT('Ctrl Pts',(-0.216988536104113,1.04302337738546,
2.92962089354545));
#25466=CARTESIAN_POINT('Ctrl Pts',(-0.216428786478487,1.04045706470233,
2.92710763990796));
#25467=CARTESIAN_POINT('Ctrl Pts',(-0.215847310465463,1.03779089346786,
2.9246182449626));
#25468=CARTESIAN_POINT('Origin',(0.,0.,3.1));
#25469=CARTESIAN_POINT('Ctrl Pts',(0.644752300229835,0.84136464826396,2.9246182449626));
#25470=CARTESIAN_POINT('Ctrl Pts',(0.646433000359351,0.843514492555987,
2.92710763990798));
#25471=CARTESIAN_POINT('Ctrl Pts',(0.648050798688572,0.845583794128261,
2.92962089354548));
#25472=CARTESIAN_POINT('Ctrl Pts',(0.655979290360836,0.85572466858529,2.94249292785856));
#25473=CARTESIAN_POINT('Ctrl Pts',(0.662318522702308,0.863831545066573,
2.95482773544112));
#25474=CARTESIAN_POINT('Ctrl Pts',(0.673252578886601,0.877812903896685,
2.98139042541308));
#25475=CARTESIAN_POINT('Ctrl Pts',(0.677847358284485,0.883687417317991,
2.9956183097423));
#25476=CARTESIAN_POINT('Ctrl Pts',(0.684755270452366,0.892518849463665,
3.02268627965537));
#25477=CARTESIAN_POINT('Ctrl Pts',(0.687704871914686,0.8962894383426,3.03802008916159));
#25478=CARTESIAN_POINT('Ctrl Pts',(0.691545075614569,0.901198384221383,
3.06935246409421));
#25479=CARTESIAN_POINT('Ctrl Pts',(0.692435660859824,0.902336752864262,
3.08535102977909));
#25480=CARTESIAN_POINT('Ctrl Pts',(0.692435660859824,0.902336752864262,
3.1));
#25481=CARTESIAN_POINT('Ctrl Pts',(0.692435660859824,0.902336752864262,
3.11464897022091));
#25482=CARTESIAN_POINT('Ctrl Pts',(0.691545075614567,0.901198384221383,
3.13064753590579));
#25483=CARTESIAN_POINT('Ctrl Pts',(0.687704871914685,0.896289438342601,
3.16197991083841));
#25484=CARTESIAN_POINT('Ctrl Pts',(0.684755270452365,0.892518849463665,
3.17731372034463));
#25485=CARTESIAN_POINT('Ctrl Pts',(0.677847358284485,0.883687417317991,
3.2043816902577));
#25486=CARTESIAN_POINT('Ctrl Pts',(0.6732525788866,0.877812903896684,3.21860957458692));
#25487=CARTESIAN_POINT('Ctrl Pts',(0.662318522702307,0.863831545066573,
3.24517226455888));
#25488=CARTESIAN_POINT('Ctrl Pts',(0.655979290360836,0.85572466858529,3.25750707214144));
#25489=CARTESIAN_POINT('Ctrl Pts',(0.648050798688553,0.845583794128237,
3.27037910645455));
#25490=CARTESIAN_POINT('Ctrl Pts',(0.646433000359339,0.843514492555969,
3.27289236009204));
#25491=CARTESIAN_POINT('Ctrl Pts',(0.644752300229836,0.841364648263959,
3.2753817550374));
#25492=CARTESIAN_POINT('Origin',(0.,0.,3.1));
#25493=CARTESIAN_POINT('',(0.447871167131128,0.589076750222415,3.2753817550374));
#25494=CARTESIAN_POINT('Origin',(0.,0.,3.2753817550374));
#25495=CARTESIAN_POINT('Ctrl Pts',(0.447871167131129,0.589076750222414,
3.2753817550374));
#25496=CARTESIAN_POINT('Ctrl Pts',(0.446194419897493,0.586923529425736,
3.27289220019637));
#25497=CARTESIAN_POINT('Ctrl Pts',(0.444580537728585,0.58485089538211,3.27037878209112));
#25498=CARTESIAN_POINT('Ctrl Pts',(0.436672122204367,0.574693882270447,
3.2575065722869));
#25499=CARTESIAN_POINT('Ctrl Pts',(0.430350710191136,0.566572846562107,
3.24517174819405));
#25500=CARTESIAN_POINT('Ctrl Pts',(0.419449625073301,0.552565269832587,
3.21860898580305));
#25501=CARTESIAN_POINT('Ctrl Pts',(0.414869876004012,0.546678794884774,
3.20438104383706));
#25502=CARTESIAN_POINT('Ctrl Pts',(0.407985330685283,0.537828888858988,
3.17731312334706));
#25503=CARTESIAN_POINT('Ctrl Pts',(0.405046225197691,0.534050030841187,
3.16197944811959));
#25504=CARTESIAN_POINT('Ctrl Pts',(0.401219893621934,0.529130146180412,
3.13064732225863));
#25505=CARTESIAN_POINT('Ctrl Pts',(0.400332631188562,0.52798915178784,3.11464887099961));
#25506=CARTESIAN_POINT('Ctrl Pts',(0.400332631188562,0.52798915178784,3.08535112900039));
#25507=CARTESIAN_POINT('Ctrl Pts',(0.401219893621934,0.529130146180412,
3.06935267774138));
#25508=CARTESIAN_POINT('Ctrl Pts',(0.405046225197691,0.534050030841187,
3.03802055188041));
#25509=CARTESIAN_POINT('Ctrl Pts',(0.407985330685283,0.537828888858988,
3.02268687665294));
#25510=CARTESIAN_POINT('Ctrl Pts',(0.414869876004012,0.546678794884774,
2.99561895616294));
#25511=CARTESIAN_POINT('Ctrl Pts',(0.419449625073304,0.552565269832584,
2.98139101419695));
#25512=CARTESIAN_POINT('Ctrl Pts',(0.430350710191138,0.566572846562104,
2.95482825180595));
#25513=CARTESIAN_POINT('Ctrl Pts',(0.436672122204369,0.574693882270445,
2.9424934277131));
#25514=CARTESIAN_POINT('Ctrl Pts',(0.444580537728587,0.584850895382108,
2.92962121790888));
#25515=CARTESIAN_POINT('Ctrl Pts',(0.446194419897493,0.586923529425736,
2.92710779980363));
#25516=CARTESIAN_POINT('Ctrl Pts',(0.447871167131129,0.589076750222414,
2.9246182449626));
#25517=CARTESIAN_POINT('Origin',(0.56114082167286,0.703648334221227,3.1));
#25518=CARTESIAN_POINT('',(0.461382453375463,0.578555297026342,3.27639564195297));
#25519=CARTESIAN_POINT('Ctrl Pts',(0.461382453375463,0.578555297026342,
3.27639564195297));
#25520=CARTESIAN_POINT('Ctrl Pts',(0.457039480081212,0.582018702657134,
3.27639564195297));
#25521=CARTESIAN_POINT('Ctrl Pts',(0.452502352671194,0.585555690407633,
3.27607258736419));
#25522=CARTESIAN_POINT('Ctrl Pts',(0.447871167131128,0.589076750222415,
3.2753817550374));
#25523=CARTESIAN_POINT('',(0.56114082167286,0.703648334221227,3.33815));
#25524=CARTESIAN_POINT('Origin',(0.56114082167286,0.703648334221227,3.1));
#25525=CARTESIAN_POINT('',(0.474646655807069,0.56772401052903,3.2753817550374));
#25526=CARTESIAN_POINT('Ctrl Pts',(0.474646655807069,0.56772401052903,3.2753817550374));
#25527=CARTESIAN_POINT('Ctrl Pts',(0.470183340581477,0.571455573060031,
3.27607258736419));
#25528=CARTESIAN_POINT('Ctrl Pts',(0.465725426669714,0.57509189139555,3.27639564195297));
#25529=CARTESIAN_POINT('Ctrl Pts',(0.461382453375463,0.578555297026342,
3.27639564195297));
#25530=CARTESIAN_POINT('Ctrl Pts',(0.474646655807069,0.56772401052903,2.9246182449626));
#25531=CARTESIAN_POINT('Ctrl Pts',(0.472920532111735,0.565610166146593,
2.92710779980363));
#25532=CARTESIAN_POINT('Ctrl Pts',(0.471258985898383,0.563575542910017,
2.92962121790888));
#25533=CARTESIAN_POINT('Ctrl Pts',(0.46311641831999,0.553605259830511,2.9424934277131));
#25534=CARTESIAN_POINT('Ctrl Pts',(0.45660564043721,0.545635238363898,2.95482825180595));
#25535=CARTESIAN_POINT('Ctrl Pts',(0.44537498254313,0.531890487153134,2.98139101419695));
#25536=CARTESIAN_POINT('Ctrl Pts',(0.440655183852335,0.526115698051596,
2.99561895616294));
#25537=CARTESIAN_POINT('Ctrl Pts',(0.433559118901799,0.517434473303403,
3.02268687665294));
#25538=CARTESIAN_POINT('Ctrl Pts',(0.430529017242168,0.513728182311292,
3.03802055188041));
#25539=CARTESIAN_POINT('Ctrl Pts',(0.426583923237528,0.508903007527151,
3.06935267774138));
#25540=CARTESIAN_POINT('Ctrl Pts',(0.425668970421903,0.507784095477554,
3.08535112900039));
#25541=CARTESIAN_POINT('Ctrl Pts',(0.425668970421903,0.507784095477554,
3.11464887099961));
#25542=CARTESIAN_POINT('Ctrl Pts',(0.426583923237527,0.508903007527151,
3.13064732225863));
#25543=CARTESIAN_POINT('Ctrl Pts',(0.430529017242168,0.513728182311292,
3.16197944811959));
#25544=CARTESIAN_POINT('Ctrl Pts',(0.433559118901799,0.517434473303403,
3.17731312334706));
#25545=CARTESIAN_POINT('Ctrl Pts',(0.440655183852335,0.526115698051596,
3.20438104383706));
#25546=CARTESIAN_POINT('Ctrl Pts',(0.445374982543131,0.531890487153134,
3.21860898580305));
#25547=CARTESIAN_POINT('Ctrl Pts',(0.456605640437211,0.545635238363898,
3.24517174819405));
#25548=CARTESIAN_POINT('Ctrl Pts',(0.463116418319992,0.553605259830509,
3.2575065722869));
#25549=CARTESIAN_POINT('Ctrl Pts',(0.471258985898385,0.563575542910015,
3.27037878209112));
#25550=CARTESIAN_POINT('Ctrl Pts',(0.472920532111735,0.565610166146593,
3.27289220019637));
#25551=CARTESIAN_POINT('Ctrl Pts',(0.474646655807069,0.56772401052903,3.2753817550374));
#25552=CARTESIAN_POINT('',(0.56114082167286,0.703648334221227,2.86185));
#25553=CARTESIAN_POINT('Origin',(0.56114082167286,0.703648334221227,3.1));
#25554=CARTESIAN_POINT('Ctrl Pts',(0.676798995897951,0.815808261267024,
3.2753817550374));
#25555=CARTESIAN_POINT('Ctrl Pts',(0.678520948142572,0.81792520809502,3.27289236009202));
#25556=CARTESIAN_POINT('Ctrl Pts',(0.680178374008934,0.819962907760957,
3.27037910645452));
#25557=CARTESIAN_POINT('Ctrl Pts',(0.688300740199246,0.829949172449061,
3.25750707214144));
#25558=CARTESIAN_POINT('Ctrl Pts',(0.694793748460268,0.837933416726651,
3.24517226455888));
#25559=CARTESIAN_POINT('Ctrl Pts',(0.705991509039914,0.851704478318938,
3.21860957458692));
#25560=CARTESIAN_POINT('Ctrl Pts',(0.710696301541893,0.8574912592173,3.2043816902577));
#25561=CARTESIAN_POINT('Ctrl Pts',(0.717769156177965,0.866191154133894,
3.17731372034463));
#25562=CARTESIAN_POINT('Ctrl Pts',(0.720788860449207,0.869905837888228,
3.16197991083841));
#25563=CARTESIAN_POINT('Ctrl Pts',(0.724720203091942,0.874742102885396,
3.13064753590579));
#25564=CARTESIAN_POINT('Ctrl Pts',(0.725631856595695,0.875863670152773,
3.11464897022091));
#25565=CARTESIAN_POINT('Ctrl Pts',(0.725631856595695,0.875863670152773,
3.1));
#25566=CARTESIAN_POINT('Ctrl Pts',(0.725631856595695,0.875863670152773,
3.08535102977909));
#25567=CARTESIAN_POINT('Ctrl Pts',(0.724720203091943,0.874742102885394,
3.06935246409421));
#25568=CARTESIAN_POINT('Ctrl Pts',(0.720788860449208,0.869905837888227,
3.03802008916159));
#25569=CARTESIAN_POINT('Ctrl Pts',(0.717769156177965,0.866191154133894,
3.02268627965537));
#25570=CARTESIAN_POINT('Ctrl Pts',(0.710696301541893,0.8574912592173,2.9956183097423));
#25571=CARTESIAN_POINT('Ctrl Pts',(0.705991509039915,0.851704478318936,
2.98139042541308));
#25572=CARTESIAN_POINT('Ctrl Pts',(0.69479374846027,0.837933416726649,2.95482773544112));
#25573=CARTESIAN_POINT('Ctrl Pts',(0.688300740199246,0.829949172449061,
2.94249292785856));
#25574=CARTESIAN_POINT('Ctrl Pts',(0.680178374008915,0.819962907760934,
2.92962089354545));
#25575=CARTESIAN_POINT('Ctrl Pts',(0.67852094814256,0.817925208095002,2.92710763990797));
#25576=CARTESIAN_POINT('Ctrl Pts',(0.676798995897952,0.815808261267023,
2.9246182449626));
#25577=CARTESIAN_POINT('Origin',(0.,0.,3.1));
#25578=CARTESIAN_POINT('',(-1.06,-1.29812560709619E-16,2.7));
#25579=CARTESIAN_POINT('',(-1.06,-1.29812560709619E-16,3.1));
#25580=CARTESIAN_POINT('Origin',(0.,0.,2.7));
#25581=CARTESIAN_POINT('Origin',(0.,0.,3.1));
#25582=CARTESIAN_POINT('Ctrl Pts',(1.05980185416667,-0.0204946311236757,
3.2753817550374));
#25583=CARTESIAN_POINT('Ctrl Pts',(1.06253056950731,-0.0205210128414943,
3.27289236009202));
#25584=CARTESIAN_POINT('Ctrl Pts',(1.06515709538297,-0.0205463556027087,
3.27037910645452));
#25585=CARTESIAN_POINT('Ctrl Pts',(1.07802888399501,-0.0206703430107339,
3.25750707214144));
#25586=CARTESIAN_POINT('Ctrl Pts',(1.08831954196908,-0.0207686864025012,
3.24517226455888));
#25587=CARTESIAN_POINT('Ctrl Pts',(1.106067880994,-0.0209373316932479,3.21860957458692));
#25588=CARTESIAN_POINT('Ctrl Pts',(1.11352555862733,-0.0210076877140537,
3.2043816902577));
#25589=CARTESIAN_POINT('Ctrl Pts',(1.12473726310291,-0.0211131723817156,
3.17731372034463));
#25590=CARTESIAN_POINT('Ctrl Pts',(1.12952427462721,-0.0211580048107555,
3.16197991083841));
#25591=CARTESIAN_POINT('Ctrl Pts',(1.13575657090491,-0.0212162903523946,
3.13064753590579));
#25592=CARTESIAN_POINT('Ctrl Pts',(1.13720185416667,-0.0212297640094256,
3.11464897022091));
#25593=CARTESIAN_POINT('Ctrl Pts',(1.13720185416667,-0.0212297640094256,
3.1));
#25594=CARTESIAN_POINT('Ctrl Pts',(1.13720185416667,-0.0212297640094256,
3.08535102977909));
#25595=CARTESIAN_POINT('Ctrl Pts',(1.13575657090491,-0.0212162903523946,
3.06935246409421));
#25596=CARTESIAN_POINT('Ctrl Pts',(1.12952427462721,-0.0211580048107555,
3.03802008916159));
#25597=CARTESIAN_POINT('Ctrl Pts',(1.12473726310291,-0.0211131723817156,
3.02268627965537));
#25598=CARTESIAN_POINT('Ctrl Pts',(1.11352555862733,-0.0210076877140537,
2.9956183097423));
#25599=CARTESIAN_POINT('Ctrl Pts',(1.106067880994,-0.0209373316932489,2.98139042541308));
#25600=CARTESIAN_POINT('Ctrl Pts',(1.08831954196908,-0.020768686402502,
2.95482773544113));
#25601=CARTESIAN_POINT('Ctrl Pts',(1.07802888399501,-0.0206703430107339,
2.94249292785856));
#25602=CARTESIAN_POINT('Ctrl Pts',(1.06515709538294,-0.0205463556027084,
2.92962089354545));
#25603=CARTESIAN_POINT('Ctrl Pts',(1.06253056950729,-0.0205210128414896,
2.92710763990796));
#25604=CARTESIAN_POINT('Ctrl Pts',(1.05980185416667,-0.0204946311236712,
2.9246182449626));
#25605=CARTESIAN_POINT('Origin',(0.,0.,3.1));
#25606=CARTESIAN_POINT('',(-0.74,-9.06238631369041E-17,3.5));
#25607=CARTESIAN_POINT('Origin',(0.,0.,3.5));
#25608=CARTESIAN_POINT('',(-0.74,-9.06238631369041E-17,3.1));
#25609=CARTESIAN_POINT('',(0.739801854166667,-0.0171235677229433,3.2753817550374));
#25610=CARTESIAN_POINT('Origin',(0.,0.,3.2753817550374));
#25611=CARTESIAN_POINT('',(0.74,-1.41339830831208E-17,3.27639564195297));
#25612=CARTESIAN_POINT('Ctrl Pts',(0.739801854166667,-0.0171235677229433,
3.2753817550374));
#25613=CARTESIAN_POINT('Ctrl Pts',(0.739936475706564,-0.0113074161803182,
3.27607258736419));
#25614=CARTESIAN_POINT('Ctrl Pts',(0.74,-0.00555487133946258,3.27639564195297));
#25615=CARTESIAN_POINT('Ctrl Pts',(0.74,-8.67361737988404E-18,3.27639564195297));
#25616=CARTESIAN_POINT('',(0.739801854166667,0.0171235677229433,3.2753817550374));
#25617=CARTESIAN_POINT('Ctrl Pts',(0.74,-8.67361737988404E-18,3.27639564195297));
#25618=CARTESIAN_POINT('Ctrl Pts',(0.74,0.0055548713394626,3.27639564195297));
#25619=CARTESIAN_POINT('Ctrl Pts',(0.739936475706564,0.0113074161803183,
3.27607258736419));
#25620=CARTESIAN_POINT('Ctrl Pts',(0.739801854166667,0.0171235677229433,
3.2753817550374));
#25621=CARTESIAN_POINT('Origin',(0.,0.,3.2753817550374));
#25622=CARTESIAN_POINT('Origin',(0.,0.,3.1));
#25623=CARTESIAN_POINT('Ctrl Pts',(0.739801854166667,-0.0171235677229416,
2.9246182449626));
#25624=CARTESIAN_POINT('Ctrl Pts',(0.737072963558652,-0.0170919902904609,
2.92710779980363));
#25625=CARTESIAN_POINT('Ctrl Pts',(0.734446273937994,-0.017061507989918,
2.92962121790888));
#25626=CARTESIAN_POINT('Ctrl Pts',(0.721574384891244,-0.0169117621307234,
2.9424934277131));
#25627=CARTESIAN_POINT('Ctrl Pts',(0.711283767580619,-0.0167906581116384,
2.95482825180595));
#25628=CARTESIAN_POINT('Ctrl Pts',(0.69353548770023,-0.0165798884102157,
2.98139101419695));
#25629=CARTESIAN_POINT('Ctrl Pts',(0.686077829425498,-0.0164903233155346,
2.99561895616294));
#25630=CARTESIAN_POINT('Ctrl Pts',(0.674866250480993,-0.0163550514337092,
3.02268687665294));
#25631=CARTESIAN_POINT('Ctrl Pts',(0.670079318016798,-0.0162968571974327,
3.03802055188041));
#25632=CARTESIAN_POINT('Ctrl Pts',(0.663847118582878,-0.0162209057734067,
3.06935267774138));
#25633=CARTESIAN_POINT('Ctrl Pts',(0.662401854166667,-0.0162031971092804,
3.08535112900039));
#25634=CARTESIAN_POINT('Ctrl Pts',(0.662401854166667,-0.0162031971092804,
3.11464887099961));
#25635=CARTESIAN_POINT('Ctrl Pts',(0.663847118582878,-0.0162209057734067,
3.13064732225863));
#25636=CARTESIAN_POINT('Ctrl Pts',(0.670079318016799,-0.0162968571974327,
3.16197944811959));
#25637=CARTESIAN_POINT('Ctrl Pts',(0.674866250480993,-0.0163550514337092,
3.17731312334706));
#25638=CARTESIAN_POINT('Ctrl Pts',(0.686077829425498,-0.0164903233155346,
3.20438104383706));
#25639=CARTESIAN_POINT('Ctrl Pts',(0.693535487700231,-0.0165798884102181,
3.21860898580305));
#25640=CARTESIAN_POINT('Ctrl Pts',(0.71128376758062,-0.0167906581116409,
3.24517174819405));
#25641=CARTESIAN_POINT('Ctrl Pts',(0.721574384891244,-0.0169117621307202,
3.2575065722869));
#25642=CARTESIAN_POINT('Ctrl Pts',(0.734446273937994,-0.0170615079899147,
3.27037878209112));
#25643=CARTESIAN_POINT('Ctrl Pts',(0.737072963558652,-0.0170919902904609,
3.27289220019637));
#25644=CARTESIAN_POINT('Ctrl Pts',(0.739801854166667,-0.0171235677229416,
3.2753817550374));
#25645=CARTESIAN_POINT('Origin',(0.9,0.,3.1));
#25646=CARTESIAN_POINT('',(0.9,-1.78583896120461E-33,2.86185));
#25647=CARTESIAN_POINT('Origin',(0.9,0.,3.1));
#25648=CARTESIAN_POINT('Ctrl Pts',(0.739801854166667,0.0171235677229416,
3.2753817550374));
#25649=CARTESIAN_POINT('Ctrl Pts',(0.737072963558652,0.0170919902904609,
3.27289220019637));
#25650=CARTESIAN_POINT('Ctrl Pts',(0.734446273937994,0.0170615079899147,
3.27037878209112));
#25651=CARTESIAN_POINT('Ctrl Pts',(0.721574384891244,0.0169117621307202,
3.2575065722869));
#25652=CARTESIAN_POINT('Ctrl Pts',(0.71128376758062,0.0167906581116409,
3.24517174819405));
#25653=CARTESIAN_POINT('Ctrl Pts',(0.693535487700231,0.0165798884102181,
3.21860898580305));
#25654=CARTESIAN_POINT('Ctrl Pts',(0.686077829425498,0.0164903233155346,
3.20438104383706));
#25655=CARTESIAN_POINT('Ctrl Pts',(0.674866250480993,0.0163550514337092,
3.17731312334706));
#25656=CARTESIAN_POINT('Ctrl Pts',(0.670079318016799,0.0162968571974327,
3.16197944811959));
#25657=CARTESIAN_POINT('Ctrl Pts',(0.663847118582878,0.0162209057734067,
3.13064732225863));
#25658=CARTESIAN_POINT('Ctrl Pts',(0.662401854166667,0.0162031971092804,
3.11464887099961));
#25659=CARTESIAN_POINT('Ctrl Pts',(0.662401854166667,0.0162031971092804,
3.08535112900039));
#25660=CARTESIAN_POINT('Ctrl Pts',(0.663847118582878,0.0162209057734067,
3.06935267774138));
#25661=CARTESIAN_POINT('Ctrl Pts',(0.670079318016798,0.0162968571974327,
3.03802055188041));
#25662=CARTESIAN_POINT('Ctrl Pts',(0.674866250480993,0.0163550514337092,
3.02268687665294));
#25663=CARTESIAN_POINT('Ctrl Pts',(0.686077829425498,0.0164903233155346,
2.99561895616294));
#25664=CARTESIAN_POINT('Ctrl Pts',(0.69353548770023,0.0165798884102157,
2.98139101419695));
#25665=CARTESIAN_POINT('Ctrl Pts',(0.711283767580619,0.0167906581116384,
2.95482825180595));
#25666=CARTESIAN_POINT('Ctrl Pts',(0.721574384891244,0.0169117621307234,
2.9424934277131));
#25667=CARTESIAN_POINT('Ctrl Pts',(0.734446273937994,0.017061507989918,
2.92962121790888));
#25668=CARTESIAN_POINT('Ctrl Pts',(0.737072963558652,0.0170919902904609,
2.92710779980363));
#25669=CARTESIAN_POINT('Ctrl Pts',(0.739801854166667,0.0171235677229416,
2.9246182449626));
#25670=CARTESIAN_POINT('',(0.9,-1.78583896120461E-33,3.33815));
#25671=CARTESIAN_POINT('Origin',(0.9,0.,3.1));
#25672=CARTESIAN_POINT('Ctrl Pts',(1.05980185416667,0.0204946311236712,
2.9246182449626));
#25673=CARTESIAN_POINT('Ctrl Pts',(1.06253056950731,0.0205210128414899,
2.92710763990798));
#25674=CARTESIAN_POINT('Ctrl Pts',(1.06515709538297,0.0205463556027087,
2.92962089354548));
#25675=CARTESIAN_POINT('Ctrl Pts',(1.07802888399501,0.0206703430107339,
2.94249292785856));
#25676=CARTESIAN_POINT('Ctrl Pts',(1.08831954196908,0.0207686864025012,
2.95482773544112));
#25677=CARTESIAN_POINT('Ctrl Pts',(1.106067880994,0.0209373316932479,2.98139042541308));
#25678=CARTESIAN_POINT('Ctrl Pts',(1.11352555862733,0.0210076877140537,
2.9956183097423));
#25679=CARTESIAN_POINT('Ctrl Pts',(1.12473726310291,0.0211131723817156,
3.02268627965537));
#25680=CARTESIAN_POINT('Ctrl Pts',(1.12952427462721,0.0211580048107574,
3.03802008916159));
#25681=CARTESIAN_POINT('Ctrl Pts',(1.13575657090491,0.0212162903523964,
3.06935246409421));
#25682=CARTESIAN_POINT('Ctrl Pts',(1.13720185416667,0.0212297640094256,
3.08535102977909));
#25683=CARTESIAN_POINT('Ctrl Pts',(1.13720185416667,0.0212297640094256,
3.1));
#25684=CARTESIAN_POINT('Ctrl Pts',(1.13720185416667,0.0212297640094256,
3.11464897022091));
#25685=CARTESIAN_POINT('Ctrl Pts',(1.13575657090491,0.0212162903523946,
3.13064753590579));
#25686=CARTESIAN_POINT('Ctrl Pts',(1.12952427462721,0.0211580048107555,
3.16197991083841));
#25687=CARTESIAN_POINT('Ctrl Pts',(1.12473726310291,0.0211131723817156,
3.17731372034463));
#25688=CARTESIAN_POINT('Ctrl Pts',(1.11352555862733,0.0210076877140537,
3.2043816902577));
#25689=CARTESIAN_POINT('Ctrl Pts',(1.106067880994,0.0209373316932487,3.21860957458692));
#25690=CARTESIAN_POINT('Ctrl Pts',(1.08831954196908,0.0207686864025019,
3.24517226455888));
#25691=CARTESIAN_POINT('Ctrl Pts',(1.07802888399501,0.0206703430107339,
3.25750707214144));
#25692=CARTESIAN_POINT('Ctrl Pts',(1.06515709538294,0.0205463556027084,
3.27037910645455));
#25693=CARTESIAN_POINT('Ctrl Pts',(1.06253056950729,0.0205210128414941,
3.27289236009204));
#25694=CARTESIAN_POINT('Ctrl Pts',(1.05980185416667,0.0204946311236757,
3.2753817550374));
#25695=CARTESIAN_POINT('Origin',(0.,0.,3.1));
#25696=CARTESIAN_POINT('Origin',(1.27,0.,2.7));
#25697=CARTESIAN_POINT('',(-1.27,-1.55530143491714E-16,2.7));
#25698=CARTESIAN_POINT('Origin',(0.,0.,2.7));
#25699=CARTESIAN_POINT('Origin',(0.,0.,2.715));
#25700=CARTESIAN_POINT('',(-1.3,-1.59204083889156E-16,2.73));
#25701=CARTESIAN_POINT('Origin',(0.,0.,2.73));
#25702=CARTESIAN_POINT('',(-1.285,-1.57367113690435E-16,2.715));
#25703=CARTESIAN_POINT('Origin',(0.,0.,3.1));
#25704=CARTESIAN_POINT('',(-1.3,-1.59204083889156E-16,3.47));
#25705=CARTESIAN_POINT('Origin',(0.,0.,3.47));
#25706=CARTESIAN_POINT('',(-1.3,-1.59204083889156E-16,3.1));
#25707=CARTESIAN_POINT('Origin',(0.,0.,3.485));
#25708=CARTESIAN_POINT('',(-1.27,-1.55530143491714E-16,3.5));
#25709=CARTESIAN_POINT('Origin',(0.,0.,3.5));
#25710=CARTESIAN_POINT('',(-1.285,-1.57367113690435E-16,3.485));
#25711=CARTESIAN_POINT('Origin',(1.06,0.,3.5));
#25712=CARTESIAN_POINT('Origin',(0.,0.,3.1));
#25713=CARTESIAN_POINT('Origin',(0.,0.,3.1));
#25714=CARTESIAN_POINT('',(-0.5,-6.12323399573677E-17,3.47));
#25715=CARTESIAN_POINT('Origin',(0.,0.,3.47));
#25716=CARTESIAN_POINT('',(-0.5,-6.12323399573677E-17,2.73));
#25717=CARTESIAN_POINT('',(-0.5,-6.12323399573677E-17,3.1));
#25718=CARTESIAN_POINT('Origin',(0.,0.,2.73));
#25719=CARTESIAN_POINT('Origin',(0.,0.,2.715));
#25720=CARTESIAN_POINT('',(-0.53,-6.49062803548097E-17,2.7));
#25721=CARTESIAN_POINT('',(-0.515,-6.30693101560887E-17,2.715));
#25722=CARTESIAN_POINT('Origin',(0.,0.,2.7));
#25723=CARTESIAN_POINT('Origin',(0.74,0.,2.7));
#25724=CARTESIAN_POINT('Origin',(0.53,0.,3.5));
#25725=CARTESIAN_POINT('',(-0.53,-6.49062803548097E-17,3.5));
#25726=CARTESIAN_POINT('Origin',(0.,0.,3.5));
#25727=CARTESIAN_POINT('Origin',(0.,0.,3.485));
#25728=CARTESIAN_POINT('',(-0.515,-6.30693101560887E-17,3.485));
#31618=UNCERTAINTY_MEASURE_WITH_UNIT(LENGTH_MEASURE(0.001),#31639,
'DISTANCE_ACCURACY_VALUE',
'Maximum model space distance between geometric entities at asserted c
onnectivities');
#31625=UNCERTAINTY_MEASURE_WITH_UNIT(LENGTH_MEASURE(0.001),#31639,
'DISTANCE_ACCURACY_VALUE',
'Maximum model space distance between geometric entities at asserted c
onnectivities');
#31631=(
GEOMETRIC_REPRESENTATION_CONTEXT(3)
GLOBAL_UNCERTAINTY_ASSIGNED_CONTEXT((#31618))
GLOBAL_UNIT_ASSIGNED_CONTEXT((#31639,#31641,#31642))
REPRESENTATION_CONTEXT('','3D')
);
#31638=(
GEOMETRIC_REPRESENTATION_CONTEXT(3)
GLOBAL_UNCERTAINTY_ASSIGNED_CONTEXT((#31625))
GLOBAL_UNIT_ASSIGNED_CONTEXT((#31639,#31641,#31642))
REPRESENTATION_CONTEXT('','3D')
);
#31639=(
LENGTH_UNIT()
NAMED_UNIT(*)
SI_UNIT(.CENTI.,.METRE.)
);
#31641=(
NAMED_UNIT(*)
PLANE_ANGLE_UNIT()
SI_UNIT($,.RADIAN.)
);
#31642=(
NAMED_UNIT(*)
SI_UNIT($,.STERADIAN.)
SOLID_ANGLE_UNIT()
);
#31648=SHAPE_DEFINITION_REPRESENTATION(#31660,#31709);
#31660=PRODUCT_DEFINITION_SHAPE('',$,#31722);
#31709=SHAPE_REPRESENTATION('',(#12986),#31631);
#31716=PRODUCT_DEFINITION_CONTEXT('part definition',#31754,'design');
#31722=PRODUCT_DEFINITION('2026-10-22-02-42-20-042',
'05_Deep_Groove_Ball_Bearing_6000-ZZ_10x26x8',#31734,#31716);
#31734=PRODUCT_DEFINITION_FORMATION('',$,#31761);
#31754=APPLICATION_CONTEXT(
'Core Data for Automotive Mechanical Design Process');
#31755=PRODUCT_CONTEXT('part definition',#31754,'mechanical');
#31761=PRODUCT('2026-10-22-02-42-20-042',
'05_Deep_Groove_Ball_Bearing_6000-ZZ_10x26x8',$,(#31755));
#31824=COLOUR_RGB('Grey',0.48,0.52,0.57);
#31825=FILL_AREA_STYLE_COLOUR('',#31824);
#31826=FILL_AREA_STYLE('',(#31825));
#31827=SURFACE_STYLE_FILL_AREA(#31826);
#31828=SURFACE_SIDE_STYLE('',(#31827));
#31829=SURFACE_STYLE_USAGE(.BOTH.,#31828);
#31830=PRESENTATION_STYLE_ASSIGNMENT((#31829));
ENDSEC;
END-ISO-10303-21;
